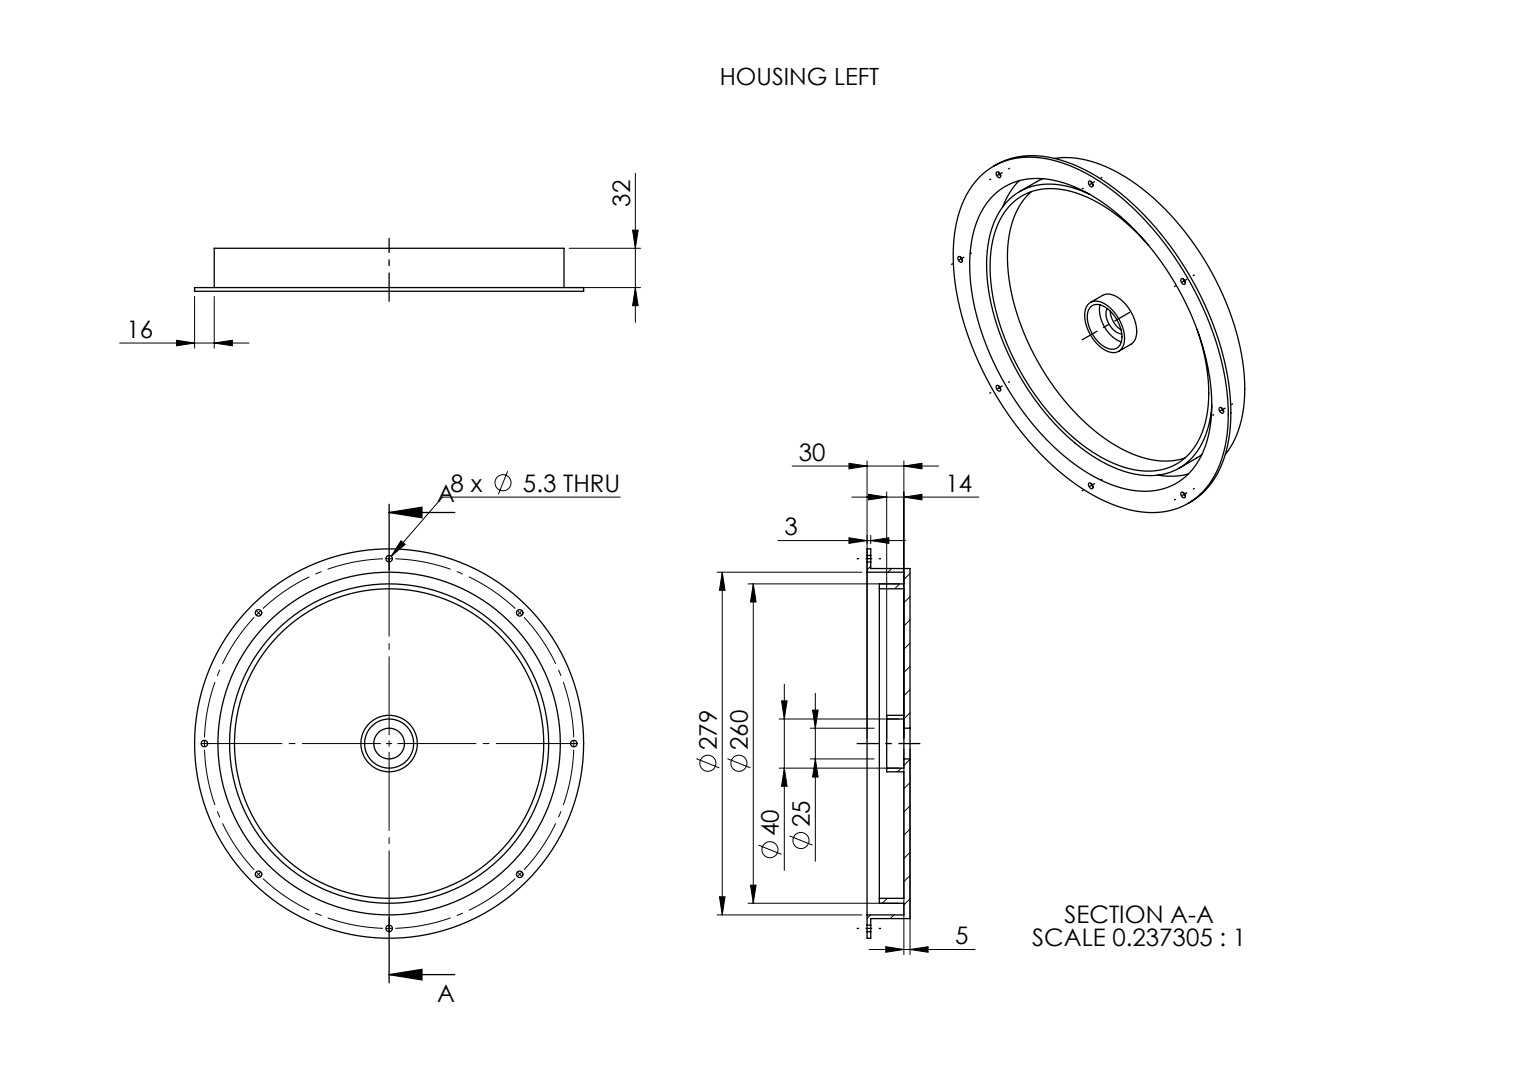
ISO-10303-21;
HEADER;
FILE_DESCRIPTION (('STEP AP214'),
    '1' );
FILE_NAME ('housing left.step',
    '2026-10-08T11:45:07',
    ( '' ),
    ( '' ),
    'SwSTEP 2.0',
    'SolidWorks 2026',
    '' );
FILE_SCHEMA (( 'AUTOMOTIVE_DESIGN' ));
ENDSEC;

DATA;
#75=EDGE_CURVE ( 'NONE', #34974, #23352, #8192, .T. ) ;
#80=DIRECTION ( 'NONE',  ( 1.000000000000000000, 0.000000000000000000, 0.000000000000000000 ) ) ;
#161=ADVANCED_FACE ( 'NONE', ( #9836 ), #29711, .F. ) ;
#175=EDGE_CURVE ( 'NONE', #28450, #28268, #33086, .T. ) ;
#184=DIRECTION ( 'NONE',  ( -0.2140725878556641593, -0.9768177553304296934, 0.000000000000000000 ) ) ;
#200=DIRECTION ( 'NONE',  ( -0.000000000000000000, -0.000000000000000000, 1.000000000000000000 ) ) ;
#245=ORIENTED_EDGE ( 'NONE', *, *, #22971, .F. ) ;
#258=DIRECTION ( 'NONE',  ( 1.000000000000000000, 0.000000000000000000, 0.000000000000000000 ) ) ;
#299=DIRECTION ( 'NONE',  ( 0.000000000000000000, 0.000000000000000000, 1.000000000000000000 ) ) ;
#312=CARTESIAN_POINT ( 'NONE',  ( -130.0000000000000284, 4.615443851143735910E-16, -20.00000000000000000 ) ) ;
#362=DIRECTION ( 'NONE',  ( 0.000000000000000000, 0.000000000000000000, 1.000000000000000000 ) ) ;
#399=CIRCLE ( 'NONE', #24866, 2.649999999999985700 ) ;
#444=EDGE_CURVE ( 'NONE', #11655, #6621, #32347, .T. ) ;
#503=PRESENTATION_STYLE_ASSIGNMENT (( #8148 ) ) ;
#513=ORIENTED_EDGE ( 'NONE', *, *, #20207, .F. ) ;
#609=ORIENTED_EDGE ( 'NONE', *, *, #444, .T. ) ;
#632=EDGE_CURVE ( 'NONE', #15962, #12068, #5869, .T. ) ;
#675=DIRECTION ( 'NONE',  ( 0.000000000000000000, 0.000000000000000000, 1.000000000000000000 ) ) ;
#711=( NAMED_UNIT ( * ) SI_UNIT ( $, .STERADIAN. ) SOLID_ANGLE_UNIT ( ) );
#788=EDGE_CURVE ( 'NONE', #6621, #11655, #5224, .T. ) ;
#808=ORIENTED_EDGE ( 'NONE', *, *, #27933, .T. ) ;
#847=FACE_BOUND ( 'NONE', #40043, .T. ) ;
#875=EDGE_LOOP ( 'NONE', ( #609, #11222 ) ) ;
#896=CARTESIAN_POINT ( 'NONE',  ( 109.0695705685763244, -106.4195705685744855, 6.999999999999998224 ) ) ;
#920=FACE_BOUND ( 'NONE', #14156, .T. ) ;
#939=CARTESIAN_POINT ( 'NONE',  ( -153.1500000000000057, -5.251434100941175950E-13, 9.999999999999998224 ) ) ;
#940=EDGE_CURVE ( 'NONE', #30306, #27122, #29838, .T. ) ;
#943=VECTOR ( 'NONE', #11137, 1000.000000000000000 ) ;
#945=CYLINDRICAL_SURFACE ( 'NONE', #19407, 126.0000000000000284 ) ;
#994=DIRECTION ( 'NONE',  ( 1.000000000000000000, 0.000000000000000000, 0.000000000000000000 ) ) ;
#1052=CARTESIAN_POINT ( 'NONE',  ( 5.657435538624008755E-15, 4.615443851143735910E-16, -20.00000000000001776 ) ) ;
#1084=CARTESIAN_POINT ( 'NONE',  ( 0.000000000000000000, 0.000000000000000000, -20.00000000000000000 ) ) ;
#1151=FACE_OUTER_BOUND ( 'NONE', #14974, .T. ) ;
#1244=AXIS2_PLACEMENT_3D ( 'NONE', #41617, #5610, #15672 ) ;
#1262=ORIENTED_EDGE ( 'NONE', *, *, #13717, .T. ) ;
#1270=DIRECTION ( 'NONE',  ( 1.000000000000000000, 0.000000000000000000, 0.000000000000000000 ) ) ;
#1292=ORIENTED_EDGE ( 'NONE', *, *, #35237, .T. ) ;
#1369=CARTESIAN_POINT ( 'NONE',  ( 106.4195705685741302, 106.4195705685767166, 6.999999999999998224 ) ) ;
#1372=( NAMED_UNIT ( * ) PLANE_ANGLE_UNIT ( ) SI_UNIT ( $, .RADIAN. ) );
#1390=DIRECTION ( 'NONE',  ( -0.000000000000000000, -0.000000000000000000, 1.000000000000000000 ) ) ;
#1393=FACE_BOUND ( 'NONE', #25323, .T. ) ;
#1394=DIRECTION ( 'NONE',  ( 1.000000000000000000, 0.000000000000000000, 0.000000000000000000 ) ) ;
#1439=ORIENTED_EDGE ( 'NONE', *, *, #28050, .T. ) ;
#1443=DIRECTION ( 'NONE',  ( 1.000000000000000000, 0.000000000000000000, 0.000000000000000000 ) ) ;
#1466=EDGE_CURVE ( 'NONE', #2965, #37680, #15217, .T. ) ;
#1475=CIRCLE ( 'NONE', #9143, 158.5000000000000284 ) ;
#1531=PRODUCT_CONTEXT ( 'NONE', #24534, 'mechanical' ) ;
#1567=CIRCLE ( 'NONE', #7140, 139.5000000000000000 ) ;
#1595=EDGE_CURVE ( 'NONE', #28016, #28450, #25874, .T. ) ;
#1638=CARTESIAN_POINT ( 'NONE',  ( 0.000000000000000000, 0.000000000000000000, 6.999999999999998224 ) ) ;
#1664=VERTEX_POINT ( 'NONE', #29142 ) ;
#1678=DIRECTION ( 'NONE',  ( 0.000000000000000000, 0.000000000000000000, 1.000000000000000000 ) ) ;
#1720=FACE_OUTER_BOUND ( 'NONE', #13675, .T. ) ;
#1744=CARTESIAN_POINT ( 'NONE',  ( 0.000000000000000000, 0.000000000000000000, -20.00000000000000000 ) ) ;
#1748=DIRECTION ( 'NONE',  ( 1.000000000000000000, 0.000000000000000000, 0.000000000000000000 ) ) ;
#1771=ORIENTED_EDGE ( 'NONE', *, *, #632, .T. ) ;
#1778=CARTESIAN_POINT ( 'NONE',  ( -139.5000000000000000, 0.000000000000000000, -20.00000000000000000 ) ) ;
#1886=CIRCLE ( 'NONE', #13069, 2.649999999999985700 ) ;
#1891=CARTESIAN_POINT ( 'NONE',  ( 0.000000000000000000, 0.000000000000000000, 6.999999999999998224 ) ) ;
#1951=AXIS2_PLACEMENT_3D ( 'NONE', #27384, #1390, #37822 ) ;
#2068=SURFACE_STYLE_USAGE ( .BOTH. , #26308 ) ;
#2083=VECTOR ( 'NONE', #34828, 1000.000000000000000 ) ;
#2084=CIRCLE ( 'NONE', #27888, 2.649999999999999467 ) ;
#2142=CARTESIAN_POINT ( 'NONE',  ( 0.000000000000000000, 0.000000000000000000, 9.999999999999998224 ) ) ;
#2145=ORIENTED_EDGE ( 'NONE', *, *, #7382, .T. ) ;
#2163=ORIENTED_EDGE ( 'NONE', *, *, #33430, .T. ) ;
#2172=AXIS2_PLACEMENT_3D ( 'NONE', #12279, #2402, #11860 ) ;
#2173=ORIENTED_EDGE ( 'NONE', *, *, #36590, .T. ) ;
#2189=ADVANCED_FACE ( 'NONE', ( #42996 ), #37911, .T. ) ;
#2226=DIRECTION ( 'NONE',  ( 1.000000000000000000, 0.000000000000000000, 0.000000000000000000 ) ) ;
#2259=DIRECTION ( 'NONE',  ( 0.000000000000000000, 0.000000000000000000, 1.000000000000000000 ) ) ;
#2305=EDGE_CURVE ( 'NONE', #20768, #38293, #28984, .T. ) ;
#2326=EDGE_LOOP ( 'NONE', ( #31321, #23179 ) ) ;
#2402=DIRECTION ( 'NONE',  ( 0.000000000000000000, 0.000000000000000000, 1.000000000000000000 ) ) ;
#2461=AXIS2_PLACEMENT_3D ( 'NONE', #39829, #23101, #19398 ) ;
#2472=CARTESIAN_POINT ( 'NONE',  ( 12.50000000000000000, 0.000000000000000000, -25.00000000000000000 ) ) ;
#2475=VERTEX_POINT ( 'NONE', #2950 ) ;
#2505=CYLINDRICAL_SURFACE ( 'NONE', #3072, 2.649999999999999467 ) ;
#2518=EDGE_CURVE ( 'NONE', #2965, #40561, #27577, .T. ) ;
#2556=LINE ( 'NONE', #43131, #13851 ) ;
#2582=VERTEX_POINT ( 'NONE', #3169 ) ;
#2584=CARTESIAN_POINT ( 'NONE',  ( 0.000000000000000000, -150.5000000000000284, 6.999999999999998224 ) ) ;
#2695=AXIS2_PLACEMENT_3D ( 'NONE', #14541, #21548, #27844 ) ;
#2713=DIRECTION ( 'NONE',  ( -0.000000000000000000, -0.000000000000000000, 1.000000000000000000 ) ) ;
#2721=ORIENTED_EDGE ( 'NONE', *, *, #75, .T. ) ;
#2788=CARTESIAN_POINT ( 'NONE',  ( 0.000000000000000000, 0.000000000000000000, 9.999999999999998224 ) ) ;
#2796=EDGE_CURVE ( 'NONE', #41293, #28005, #41533, .T. ) ;
#2831=DIRECTION ( 'NONE',  ( 1.000000000000000000, 0.000000000000000000, 0.000000000000000000 ) ) ;
#2877=DIRECTION ( 'NONE',  ( 1.000000000000000000, 0.000000000000000000, 0.000000000000000000 ) ) ;
#2904=DIRECTION ( 'NONE',  ( -0.000000000000000000, -0.000000000000000000, -1.000000000000000000 ) ) ;
#2926=CARTESIAN_POINT ( 'NONE',  ( 5.657435538624008755E-15, 4.615443851143735910E-16, 0.000000000000000000 ) ) ;
#2950=CARTESIAN_POINT ( 'NONE',  ( -109.0695705685756138, 106.4195705685752529, 6.999999999999998224 ) ) ;
#2965=VERTEX_POINT ( 'NONE', #39777 ) ;
#3029=FACE_OUTER_BOUND ( 'NONE', #8660, .T. ) ;
#3052=ADVANCED_BREP_SHAPE_REPRESENTATION ( '', ( #27661, #13552 ), #23961 ) ;
#3072=AXIS2_PLACEMENT_3D ( 'NONE', #19367, #2713, #18954 ) ;
#3088=ORIENTED_EDGE ( 'NONE', *, *, #34298, .T. ) ;
#3108=CARTESIAN_POINT ( 'NONE',  ( 150.5000000000000284, 1.576403824487674918E-12, 10.00000000000000000 ) ) ;
#3164=VERTEX_POINT ( 'NONE', #40215 ) ;
#3166=AXIS2_PLACEMENT_3D ( 'NONE', #30269, #27218, #33093 ) ;
#3169=CARTESIAN_POINT ( 'NONE',  ( 103.7695705685763556, -106.4195705685744855, 6.999999999999998224 ) ) ;
#3225=LINE ( 'NONE', #33785, #10904 ) ;
#3240=AXIS2_PLACEMENT_3D ( 'NONE', #12229, #24926, #42295 ) ;
#3260=CIRCLE ( 'NONE', #40212, 12.50000000000000000 ) ;
#3276=CARTESIAN_POINT ( 'NONE',  ( 126.0000000000000284, 1.589209405437102375E-14, -20.00000000000001776 ) ) ;
#3294=VECTOR ( 'NONE', #28045, 1000.000000000000000 ) ;
#3361=ORIENTED_EDGE ( 'NONE', *, *, #28288, .F. ) ;
#3447=VECTOR ( 'NONE', #13140, 1000.000000000000000 ) ;
#3488=FACE_OUTER_BOUND ( 'NONE', #19442, .T. ) ;
#3546=ORIENTED_EDGE ( 'NONE', *, *, #10588, .T. ) ;
#3569=VERTEX_POINT ( 'NONE', #20806 ) ;
#3594=CIRCLE ( 'NONE', #22478, 2.649999999999999467 ) ;
#3655=DIRECTION ( 'NONE',  ( 1.000000000000000000, 0.000000000000000000, 0.000000000000000000 ) ) ;
#3671=EDGE_LOOP ( 'NONE', ( #19488, #23768 ) ) ;
#3694=CARTESIAN_POINT ( 'NONE',  ( -150.5000000000000284, -5.254679414958916394E-13, 10.00000000000000000 ) ) ;
#3761=ORIENTED_EDGE ( 'NONE', *, *, #2518, .F. ) ;
#3767=DIRECTION ( 'NONE',  ( -0.000000000000000000, -0.000000000000000000, -1.000000000000000000 ) ) ;
#3782=DIRECTION ( 'NONE',  ( 0.000000000000000000, 0.000000000000000000, 1.000000000000000000 ) ) ;
#3821=AXIS2_PLACEMENT_3D ( 'NONE', #37877, #7998, #1443 ) ;
#3852=CARTESIAN_POINT ( 'NONE',  ( 0.000000000000000000, 0.000000000000000000, 0.000000000000000000 ) ) ;
#3942=VERTEX_POINT ( 'NONE', #32718 ) ;
#3945=CIRCLE ( 'NONE', #31183, 2.649999999999985700 ) ;
#3986=( NAMED_UNIT ( * ) SI_UNIT ( $, .STERADIAN. ) SOLID_ANGLE_UNIT ( ) );
#4187=EDGE_LOOP ( 'NONE', ( #28475, #30183, #13933, #34459 ) ) ;
#4292=CIRCLE ( 'NONE', #21782, 2.649999999999985700 ) ;
#4298=ORIENTED_EDGE ( 'NONE', *, *, #28288, .T. ) ;
#4317=CIRCLE ( 'NONE', #7824, 130.0000000000000284 ) ;
#4372=CARTESIAN_POINT ( 'NONE',  ( 150.5000000000000284, 1.576403824487674918E-12, 9.999999999999998224 ) ) ;
#4387=CARTESIAN_POINT ( 'NONE',  ( 0.000000000000000000, 0.000000000000000000, 9.999999999999998224 ) ) ;
#4555=CIRCLE ( 'NONE', #28979, 20.00000000000000000 ) ;
#4619=CARTESIAN_POINT ( 'NONE',  ( -2.649999999999987477, 150.5000000000000284, 10.00000000000000000 ) ) ;
#4648=( LENGTH_UNIT ( ) NAMED_UNIT ( * ) SI_UNIT ( .MILLI., .METRE. ) );
#4682=DIRECTION ( 'NONE',  ( -0.000000000000000000, -0.000000000000000000, 1.000000000000000000 ) ) ;
#4770=CARTESIAN_POINT ( 'NONE',  ( -103.7695705685756025, 106.4195705685752529, 6.999999999999998224 ) ) ;
#4831=CARTESIAN_POINT ( 'NONE',  ( 0.000000000000000000, 0.000000000000000000, -6.000000000000000000 ) ) ;
#4867=CARTESIAN_POINT ( 'NONE',  ( 0.000000000000000000, 0.000000000000000000, -25.00000000000000000 ) ) ;
#4995=DIRECTION ( 'NONE',  ( 0.000000000000000000, 0.000000000000000000, 1.000000000000000000 ) ) ;
#5016=VERTEX_POINT ( 'NONE', #15220 ) ;
#5024=AXIS2_PLACEMENT_3D ( 'NONE', #1084, #17511, #38393 ) ;
#5098=CYLINDRICAL_SURFACE ( 'NONE', #13103, 130.0000000000000284 ) ;
#5119=LINE ( 'NONE', #18713, #39076 ) ;
#5134=DIRECTION ( 'NONE',  ( 1.000000000000000000, 0.000000000000000000, 0.000000000000000000 ) ) ;
#5179=ORIENTED_EDGE ( 'NONE', *, *, #33784, .F. ) ;
#5213=VERTEX_POINT ( 'NONE', #39137 ) ;
#5224=CIRCLE ( 'NONE', #8679, 2.649999999999985700 ) ;
#5317=LINE ( 'NONE', #21528, #42896 ) ;
#5345=DIRECTION ( 'NONE',  ( -0.000000000000000000, -0.000000000000000000, 1.000000000000000000 ) ) ;
#5391=ORIENTED_EDGE ( 'NONE', *, *, #27933, .F. ) ;
#5468=ADVANCED_FACE ( 'NONE', ( #920, #8146 ), #40627, .F. ) ;
#5476=AXIS2_PLACEMENT_3D ( 'NONE', #21855, #25543, #42061 ) ;
#5493=ADVANCED_FACE ( 'NONE', ( #1151 ), #28023, .F. ) ;
#5594=PLANE ( 'NONE',  #34929 ) ;
#5610=DIRECTION ( 'NONE',  ( 0.000000000000000000, 0.000000000000000000, 1.000000000000000000 ) ) ;
#5644=DIRECTION ( 'NONE',  ( -1.000000000000000000, 0.000000000000000000, 0.000000000000000000 ) ) ;
#5674=ORIENTED_EDGE ( 'NONE', *, *, #18541, .F. ) ;
#5739=FACE_OUTER_BOUND ( 'NONE', #17879, .T. ) ;
#5869=CIRCLE ( 'NONE', #35146, 2.649999999999985700 ) ;
#5893=CIRCLE ( 'NONE', #40701, 2.649999999999985700 ) ;
#6004=AXIS2_PLACEMENT_3D ( 'NONE', #35091, #41640, #25530 ) ;
#6057=EDGE_LOOP ( 'NONE', ( #5391, #29218, #14335, #40689 ) ) ;
#6137=VECTOR ( 'NONE', #38491, 1000.000000000000000 ) ;
#6207=LINE ( 'NONE', #19553, #14969 ) ;
#6217=EDGE_CURVE ( 'NONE', #3164, #32065, #39038, .T. ) ;
#6364=EDGE_LOOP ( 'NONE', ( #10639, #808, #37020, #513 ) ) ;
#6427=DIRECTION ( 'NONE',  ( -0.000000000000000000, -0.000000000000000000, -1.000000000000000000 ) ) ;
#6507=ORIENTED_EDGE ( 'NONE', *, *, #22971, .T. ) ;
#6621=VERTEX_POINT ( 'NONE', #17369 ) ;
#6654=CARTESIAN_POINT ( 'NONE',  ( 0.000000000000000000, 0.000000000000000000, -20.00000000000000000 ) ) ;
#6679=ORIENTED_EDGE ( 'NONE', *, *, #36590, .F. ) ;
#6720=ADVANCED_FACE ( 'NONE', ( #27590 ), #15166, .F. ) ;
#6743=CIRCLE ( 'NONE', #30462, 158.5000000000000284 ) ;
#6764=DIRECTION ( 'NONE',  ( 1.000000000000000000, 0.000000000000000000, 0.000000000000000000 ) ) ;
#6777=AXIS2_PLACEMENT_3D ( 'NONE', #12751, #29978, #2877 ) ;
#6785=DIRECTION ( 'NONE',  ( 0.000000000000000000, 0.000000000000000000, 1.000000000000000000 ) ) ;
#6787=PLANE ( 'NONE',  #10176 ) ;
#6910=ADVANCED_FACE ( 'NONE', ( #9212 ), #18676, .F. ) ;
#6987=CARTESIAN_POINT ( 'NONE',  ( 20.00000000000000000, 2.449293598294706513E-15, -20.00000000000000000 ) ) ;
#7016=EDGE_LOOP ( 'NONE', ( #20071, #3761, #31295, #27188 ) ) ;
#7018=CARTESIAN_POINT ( 'NONE',  ( 5.657435538624008755E-15, 4.615443851143735910E-16, 367.6955262170047263 ) ) ;
#7051=CARTESIAN_POINT ( 'NONE',  ( 126.0000000000000284, 1.589209405437102375E-14, 0.000000000000000000 ) ) ;
#7076=CARTESIAN_POINT ( 'NONE',  ( 0.000000000000000000, 0.000000000000000000, -20.00000000000000000 ) ) ;
#7140=AXIS2_PLACEMENT_3D ( 'NONE', #1744, #8084, #37747 ) ;
#7184=CARTESIAN_POINT ( 'NONE',  ( 0.000000000000000000, 0.000000000000000000, -25.00000000000000000 ) ) ;
#7230=CYLINDRICAL_SURFACE ( 'NONE', #42624, 12.50000000000000000 ) ;
#7288=DIRECTION ( 'NONE',  ( 0.000000000000000000, 0.000000000000000000, 1.000000000000000000 ) ) ;
#7324=AXIS2_PLACEMENT_3D ( 'NONE', #19545, #16050, #19335 ) ;
#7325=EDGE_LOOP ( 'NONE', ( #19158, #18409 ) ) ;
#7345=ORIENTED_EDGE ( 'NONE', *, *, #16067, .T. ) ;
#7349=EDGE_CURVE ( 'NONE', #2475, #5016, #19890, .T. ) ;
#7365=AXIS2_PLACEMENT_3D ( 'NONE', #33738, #23312, #43123 ) ;
#7382=EDGE_CURVE ( 'NONE', #38293, #23352, #26309, .T. ) ;
#7412=EDGE_LOOP ( 'NONE', ( #17057, #36600 ) ) ;
#7425=CARTESIAN_POINT ( 'NONE',  ( 2.649999999999987477, -150.5000000000000284, 10.00000000000000000 ) ) ;
#7434=AXIS2_PLACEMENT_3D ( 'NONE', #40284, #29687, #25987 ) ;
#7471=DIRECTION ( 'NONE',  ( 0.000000000000000000, 0.000000000000000000, 1.000000000000000000 ) ) ;
#7474=ORIENTED_EDGE ( 'NONE', *, *, #25003, .T. ) ;
#7531=EDGE_LOOP ( 'NONE', ( #41415, #27687, #7686, #2145 ) ) ;
#7538=CARTESIAN_POINT ( 'NONE',  ( 147.8500000000000227, 1.576728355889448963E-12, 10.00000000000000000 ) ) ;
#7557=CIRCLE ( 'NONE', #26359, 2.649999999999993694 ) ;
#7686=ORIENTED_EDGE ( 'NONE', *, *, #2305, .T. ) ;
#7694=ORIENTED_EDGE ( 'NONE', *, *, #14997, .F. ) ;
#7706=LINE ( 'NONE', #10554, #42197 ) ;
#7709=( NAMED_UNIT ( * ) PLANE_ANGLE_UNIT ( ) SI_UNIT ( $, .RADIAN. ) );
#7723=DIRECTION ( 'NONE',  ( -0.000000000000000000, -0.000000000000000000, -1.000000000000000000 ) ) ;
#7724=DIRECTION ( 'NONE',  ( 1.000000000000000000, 0.000000000000000000, 0.000000000000000000 ) ) ;
#7728=DIRECTION ( 'NONE',  ( -0.000000000000000000, -0.000000000000000000, -1.000000000000000000 ) ) ;
#7731=AXIS2_PLACEMENT_3D ( 'NONE', #19976, #10765, #37371 ) ;
#7745=DIRECTION ( 'NONE',  ( -1.000000000000000000, 0.000000000000000000, 0.000000000000000000 ) ) ;
#7824=AXIS2_PLACEMENT_3D ( 'NONE', #33782, #29898, #3655 ) ;
#7826=VERTEX_POINT ( 'NONE', #9568 ) ;
#7842=DIRECTION ( 'NONE',  ( -0.2140725878556641315, -0.9768177553304295824, 0.000000000000000000 ) ) ;
#7908=AXIS2_PLACEMENT_3D ( 'NONE', #29094, #22149, #16213 ) ;
#7914=DIRECTION ( 'NONE',  ( 0.000000000000000000, 0.000000000000000000, 1.000000000000000000 ) ) ;
#7943=DIRECTION ( 'NONE',  ( 0.000000000000000000, 0.000000000000000000, 1.000000000000000000 ) ) ;
#7998=DIRECTION ( 'NONE',  ( -0.000000000000000000, -0.000000000000000000, 1.000000000000000000 ) ) ;
#8081=PLANE ( 'NONE',  #5024 ) ;
#8084=DIRECTION ( 'NONE',  ( -0.000000000000000000, -0.000000000000000000, -1.000000000000000000 ) ) ;
#8090=CARTESIAN_POINT ( 'NONE',  ( 106.4195705685763471, -106.4195705685744855, 10.00000000000000000 ) ) ;
#8146=FACE_OUTER_BOUND ( 'NONE', #40371, .T. ) ;
#8148=SURFACE_STYLE_USAGE ( .BOTH. , #11433 ) ;
#8184=DIRECTION ( 'NONE',  ( -0.000000000000000000, -0.000000000000000000, -1.000000000000000000 ) ) ;
#8192=LINE ( 'NONE', #22547, #31702 ) ;
#8209=EDGE_CURVE ( 'NONE', #11655, #16140, #8235, .T. ) ;
#8223=CARTESIAN_POINT ( 'NONE',  ( 103.7695705685741387, 106.4195705685767166, 9.999999999999998224 ) ) ;
#8231=DIRECTION ( 'NONE',  ( -0.000000000000000000, -0.000000000000000000, 1.000000000000000000 ) ) ;
#8235=LINE ( 'NONE', #11750, #32805 ) ;
#8264=CYLINDRICAL_SURFACE ( 'NONE', #32930, 23.00000000000000000 ) ;
#8293=ORIENTED_EDGE ( 'NONE', *, *, #8555, .T. ) ;
#8307=ADVANCED_FACE ( 'NONE', ( #36115, #22864, #25905, #35681, #19369, #42866, #38957, #15649, #19576, #12381 ), #5594, .T. ) ;
#8310=SHAPE_DEFINITION_REPRESENTATION ( #9548, #39082 ) ;
#8349=ORIENTED_EDGE ( 'NONE', *, *, #30164, .T. ) ;
#8374=EDGE_CURVE ( 'NONE', #37517, #41239, #41167, .T. ) ;
#8432=VERTEX_POINT ( 'NONE', #9927 ) ;
#8469=DIRECTION ( 'NONE',  ( -1.000000000000000000, 0.000000000000000000, 0.000000000000000000 ) ) ;
#8490=FACE_OUTER_BOUND ( 'NONE', #6364, .T. ) ;
#8517=VECTOR ( 'NONE', #35103, 1000.000000000000000 ) ;
#8533=EDGE_LOOP ( 'NONE', ( #21293, #11741, #40964, #39910 ) ) ;
#8551=ORIENTED_EDGE ( 'NONE', *, *, #788, .F. ) ;
#8555=EDGE_CURVE ( 'NONE', #19787, #10716, #29372, .T. ) ;
#8565=ORIENTED_EDGE ( 'NONE', *, *, #34904, .F. ) ;
#8660=EDGE_LOOP ( 'NONE', ( #33670, #37022, #26076, #245 ) ) ;
#8679=AXIS2_PLACEMENT_3D ( 'NONE', #29666, #42940, #26395 ) ;
#8796=EDGE_CURVE ( 'NONE', #38324, #36435, #4292, .T. ) ;
#8830=ORIENTED_EDGE ( 'NONE', *, *, #24249, .T. ) ;
#8839=EDGE_LOOP ( 'NONE', ( #40459, #2721, #35422, #10366 ) ) ;
#8852=CIRCLE ( 'NONE', #3240, 2.649999999999987477 ) ;
#8879=ORIENTED_EDGE ( 'NONE', *, *, #36479, .F. ) ;
#8905=VECTOR ( 'NONE', #17273, 1000.000000000000000 ) ;
#8919=PLANE ( 'NONE',  #35283 ) ;
#8933=LINE ( 'NONE', #32060, #8517 ) ;
#8965=EDGE_CURVE ( 'NONE', #2475, #25511, #3594, .T. ) ;
#8993=CIRCLE ( 'NONE', #16692, 139.5000000000000000 ) ;
#9035=EDGE_LOOP ( 'NONE', ( #8293, #8349 ) ) ;
#9037=EDGE_CURVE ( 'NONE', #22117, #28268, #8933, .T. ) ;
#9039=FACE_BOUND ( 'NONE', #21670, .T. ) ;
#9141=FACE_OUTER_BOUND ( 'NONE', #42367, .T. ) ;
#9143=AXIS2_PLACEMENT_3D ( 'NONE', #2788, #12871, #22502 ) ;
#9146=DIRECTION ( 'NONE',  ( 1.000000000000000000, 0.000000000000000000, 0.000000000000000000 ) ) ;
#9170=AXIS2_PLACEMENT_3D ( 'NONE', #24435, #11320, #23998 ) ;
#9175=CARTESIAN_POINT ( 'NONE',  ( 0.000000000000000000, 150.5000000000000284, 10.00000000000000000 ) ) ;
#9185=DIRECTION ( 'NONE',  ( 1.000000000000000000, 0.000000000000000000, 0.000000000000000000 ) ) ;
#9212=FACE_OUTER_BOUND ( 'NONE', #26209, .T. ) ;
#9242=FACE_OUTER_BOUND ( 'NONE', #8839, .T. ) ;
#9269=VERTEX_POINT ( 'NONE', #32695 ) ;
#9270=DIRECTION ( 'NONE',  ( -0.000000000000000000, -0.000000000000000000, 1.000000000000000000 ) ) ;
#9272=EDGE_CURVE ( 'NONE', #37517, #39291, #36171, .T. ) ;
#9380=CARTESIAN_POINT ( 'NONE',  ( -109.0695705685756138, 106.4195705685752529, 9.999999999999998224 ) ) ;
#9431=VECTOR ( 'NONE', #11247, 1000.000000000000000 ) ;
#9476=LINE ( 'NONE', #2472, #27599 ) ;
#9490=EDGE_CURVE ( 'NONE', #12068, #15962, #25975, .T. ) ;
#9509=CARTESIAN_POINT ( 'NONE',  ( -2.649999999999993694, 150.5000000000000284, 6.999999999999998224 ) ) ;
#9548=PRODUCT_DEFINITION_SHAPE ( 'NONE', 'NONE',  #35852 ) ;
#9556=LINE ( 'NONE', #15917, #18343 ) ;
#9561=AXIS2_PLACEMENT_3D ( 'NONE', #22432, #41811, #11958 ) ;
#9568=CARTESIAN_POINT ( 'NONE',  ( 23.00000000000000000, 2.816687638038912352E-15, -6.000000000000000000 ) ) ;
#9596=CARTESIAN_POINT ( 'NONE',  ( 0.000000000000000000, -150.5000000000000284, 9.999999999999998224 ) ) ;
#9620=AXIS2_PLACEMENT_3D ( 'NONE', #7076, #10578, #31307 ) ;
#9670=ADVANCED_FACE ( 'NONE', ( #34629 ), #24424, .T. ) ;
#9800=DIRECTION ( 'NONE',  ( 1.000000000000000000, 0.000000000000000000, 0.000000000000000000 ) ) ;
#9823=EDGE_LOOP ( 'NONE', ( #26961, #29977, #17627, #22621 ) ) ;
#9836=FACE_OUTER_BOUND ( 'NONE', #31839, .T. ) ;
#9927=CARTESIAN_POINT ( 'NONE',  ( 103.7695705685741387, 106.4195705685767166, 6.999999999999998224 ) ) ;
#9959=ORIENTED_EDGE ( 'NONE', *, *, #12072, .T. ) ;
#10001=MECHANICAL_DESIGN_GEOMETRIC_PRESENTATION_REPRESENTATION('',(#17715),#37156);
#10052=DIRECTION ( 'NONE',  ( 1.000000000000000000, 0.000000000000000000, 0.000000000000000000 ) ) ;
#10176=AXIS2_PLACEMENT_3D ( 'NONE', #17306, #40366, #40147 ) ;
#10213=DIRECTION ( 'NONE',  ( 1.000000000000000000, 0.000000000000000000, 0.000000000000000000 ) ) ;
#10250=LINE ( 'NONE', #30766, #39930 ) ;
#10264=CARTESIAN_POINT ( 'NONE',  ( -139.5000000000000000, 0.000000000000000000, 9.999999999999998224 ) ) ;
#10328=ORIENTED_EDGE ( 'NONE', *, *, #15054, .F. ) ;
#10366=ORIENTED_EDGE ( 'NONE', *, *, #2305, .F. ) ;
#10496=FACE_OUTER_BOUND ( 'NONE', #39299, .T. ) ;
#10523=ORIENTED_EDGE ( 'NONE', *, *, #13430, .F. ) ;
#10551=VECTOR ( 'NONE', #35339, 1000.000000000000000 ) ;
#10554=CARTESIAN_POINT ( 'NONE',  ( 158.5000000000000284, 0.000000000000000000, 6.999999999999998224 ) ) ;
#10558=FILL_AREA_STYLE_COLOUR ( '', #23278 ) ;
#10578=DIRECTION ( 'NONE',  ( 0.000000000000000000, 0.000000000000000000, 1.000000000000000000 ) ) ;
#10588=EDGE_CURVE ( 'NONE', #36784, #9269, #30759, .T. ) ;
#10615=ORIENTED_EDGE ( 'NONE', *, *, #16067, .F. ) ;
#10639=ORIENTED_EDGE ( 'NONE', *, *, #9490, .F. ) ;
#10681=LINE ( 'NONE', #27719, #8905 ) ;
#10696=CARTESIAN_POINT ( 'NONE',  ( 153.1500000000000057, 1.576403824487674918E-12, 10.00000000000000000 ) ) ;
#10699=DIRECTION ( 'NONE',  ( -0.000000000000000000, -0.000000000000000000, -1.000000000000000000 ) ) ;
#10704=ORIENTED_EDGE ( 'NONE', *, *, #11733, .F. ) ;
#10716=VERTEX_POINT ( 'NONE', #6987 ) ;
#10765=DIRECTION ( 'NONE',  ( 0.000000000000000000, 0.000000000000000000, 1.000000000000000000 ) ) ;
#10767=ORIENTED_EDGE ( 'NONE', *, *, #37473, .T. ) ;
#10786=CARTESIAN_POINT ( 'NONE',  ( -103.7695705685756167, 106.4195705685752529, 10.00000000000000000 ) ) ;
#10817=VECTOR ( 'NONE', #38137, 1000.000000000000000 ) ;
#10904=VECTOR ( 'NONE', #23355, 1000.000000000000000 ) ;
#10917=ORIENTED_EDGE ( 'NONE', *, *, #40006, .F. ) ;
#10938=DIRECTION ( 'NONE',  ( 1.000000000000000000, 0.000000000000000000, 0.000000000000000000 ) ) ;
#10945=AXIS2_PLACEMENT_3D ( 'NONE', #7018, #43017, #13825 ) ;
#10979=AXIS2_PLACEMENT_3D ( 'NONE', #21319, #4682, #21753 ) ;
#11137=DIRECTION ( 'NONE',  ( -0.000000000000000000, -0.000000000000000000, 1.000000000000000000 ) ) ;
#11150=FACE_OUTER_BOUND ( 'NONE', #25415, .T. ) ;
#11185=AXIS2_PLACEMENT_3D ( 'NONE', #9175, #26202, #39051 ) ;
#11222=ORIENTED_EDGE ( 'NONE', *, *, #788, .T. ) ;
#11237=ORIENTED_EDGE ( 'NONE', *, *, #175, .F. ) ;
#11247=DIRECTION ( 'NONE',  ( -0.000000000000000000, -0.000000000000000000, -1.000000000000000000 ) ) ;
#11261=VERTEX_POINT ( 'NONE', #36988 ) ;
#11281=CARTESIAN_POINT ( 'NONE',  ( -2.649999999999987477, -150.5000000000000284, 10.00000000000000000 ) ) ;
#11301=AXIS2_PLACEMENT_3D ( 'NONE', #3694, #17072, #10052 ) ;
#11320=DIRECTION ( 'NONE',  ( 0.000000000000000000, 0.000000000000000000, 1.000000000000000000 ) ) ;
#11362=DIRECTION ( 'NONE',  ( 0.000000000000000000, 0.000000000000000000, 1.000000000000000000 ) ) ;
#11371=AXIS2_PLACEMENT_3D ( 'NONE', #9596, #36190, #22085 ) ;
#11433=SURFACE_SIDE_STYLE ('',( #37593 ) ) ;
#11455=ORIENTED_EDGE ( 'NONE', *, *, #8374, .T. ) ;
#11467=CYLINDRICAL_SURFACE ( 'NONE', #39639, 139.5000000000000000 ) ;
#11487=ORIENTED_EDGE ( 'NONE', *, *, #40914, .T. ) ;
#11561=CIRCLE ( 'NONE', #17149, 2.649999999999985700 ) ;
#11614=ADVANCED_FACE ( 'NONE', ( #23856 ), #7230, .F. ) ;
#11655=VERTEX_POINT ( 'NONE', #15338 ) ;
#11671=DIRECTION ( 'NONE',  ( -0.000000000000000000, -0.000000000000000000, 1.000000000000000000 ) ) ;
#11684=PLANE ( 'NONE',  #13759 ) ;
#11691=DIRECTION ( 'NONE',  ( -0.000000000000000000, -0.000000000000000000, 1.000000000000000000 ) ) ;
#11733=EDGE_CURVE ( 'NONE', #6621, #39372, #9556, .T. ) ;
#11737=ADVANCED_FACE ( 'NONE', ( #22471 ), #22911, .F. ) ;
#11740=AXIS2_PLACEMENT_3D ( 'NONE', #4867, #14501, #21510 ) ;
#11741=ORIENTED_EDGE ( 'NONE', *, *, #40550, .T. ) ;
#11750=CARTESIAN_POINT ( 'NONE',  ( 153.1500000000000057, 1.576403824487674918E-12, 9.999999999999998224 ) ) ;
#11860=DIRECTION ( 'NONE',  ( 1.000000000000000000, 0.000000000000000000, 0.000000000000000000 ) ) ;
#11893=ORIENTED_EDGE ( 'NONE', *, *, #16787, .T. ) ;
#11958=DIRECTION ( 'NONE',  ( 1.000000000000000000, 0.000000000000000000, 0.000000000000000000 ) ) ;
#11999=FACE_BOUND ( 'NONE', #2326, .T. ) ;
#12011=DIRECTION ( 'NONE',  ( -0.000000000000000000, -0.000000000000000000, 1.000000000000000000 ) ) ;
#12068=VERTEX_POINT ( 'NONE', #41797 ) ;
#12072=EDGE_CURVE ( 'NONE', #8432, #38324, #21359, .T. ) ;
#12100=EDGE_CURVE ( 'NONE', #39291, #24752, #22323, .T. ) ;
#12107=DIRECTION ( 'NONE',  ( 1.000000000000000000, 0.000000000000000000, -0.000000000000000000 ) ) ;
#12136=DIRECTION ( 'NONE',  ( 0.000000000000000000, 0.000000000000000000, 1.000000000000000000 ) ) ;
#12163=DIRECTION ( 'NONE',  ( 1.000000000000000000, 0.000000000000000000, -0.000000000000000000 ) ) ;
#12166=AXIS2_PLACEMENT_3D ( 'NONE', #15515, #21655, #9146 ) ;
#12229=CARTESIAN_POINT ( 'NONE',  ( 0.000000000000000000, -150.5000000000000284, 10.00000000000000000 ) ) ;
#12247=AXIS2_PLACEMENT_3D ( 'NONE', #41980, #2259, #42188 ) ;
#12268=ORIENTED_EDGE ( 'NONE', *, *, #33800, .T. ) ;
#12273=ORIENTED_EDGE ( 'NONE', *, *, #16870, .T. ) ;
#12279=CARTESIAN_POINT ( 'NONE',  ( 0.000000000000000000, 0.000000000000000000, -20.00000000000000000 ) ) ;
#12318=DIRECTION ( 'NONE',  ( 0.000000000000000000, 0.000000000000000000, 1.000000000000000000 ) ) ;
#12329=ORIENTED_EDGE ( 'NONE', *, *, #37504, .T. ) ;
#12340=FACE_BOUND ( 'NONE', #37292, .T. ) ;
#12381=FACE_OUTER_BOUND ( 'NONE', #16135, .T. ) ;
#12426=ORIENTED_EDGE ( 'NONE', *, *, #11733, .T. ) ;
#12427=DIRECTION ( 'NONE',  ( 1.000000000000000000, 0.000000000000000000, -0.000000000000000000 ) ) ;
#12488=DIRECTION ( 'NONE',  ( -0.000000000000000000, -0.000000000000000000, -1.000000000000000000 ) ) ;
#12516=ORIENTED_EDGE ( 'NONE', *, *, #1595, .F. ) ;
#12652=AXIS2_PLACEMENT_3D ( 'NONE', #2584, #42513, #25966 ) ;
#12657=EDGE_LOOP ( 'NONE', ( #41920, #30224 ) ) ;
#12695=ORIENTED_EDGE ( 'NONE', *, *, #9272, .F. ) ;
#12728=ORIENTED_EDGE ( 'NONE', *, *, #41786, .T. ) ;
#12751=CARTESIAN_POINT ( 'NONE',  ( 0.000000000000000000, 150.5000000000000284, 9.999999999999998224 ) ) ;
#12781=LINE ( 'NONE', #39149, #26911 ) ;
#12836=AXIS2_PLACEMENT_3D ( 'NONE', #25553, #38176, #21649 ) ;
#12871=DIRECTION ( 'NONE',  ( 0.000000000000000000, 0.000000000000000000, 1.000000000000000000 ) ) ;
#13005=FILL_AREA_STYLE ('',( #38725 ) ) ;
#13069=AXIS2_PLACEMENT_3D ( 'NONE', #32531, #35774, #9185 ) ;
#13091=ORIENTED_EDGE ( 'NONE', *, *, #13893, .F. ) ;
#13103=AXIS2_PLACEMENT_3D ( 'NONE', #35620, #15591, #38902 ) ;
#13134=AXIS2_PLACEMENT_3D ( 'NONE', #7184, #20542, #6764 ) ;
#13140=DIRECTION ( 'NONE',  ( -0.000000000000000000, -0.000000000000000000, -1.000000000000000000 ) ) ;
#13185=ORIENTED_EDGE ( 'NONE', *, *, #24368, .T. ) ;
#13309=DIRECTION ( 'NONE',  ( -0.000000000000000000, -0.000000000000000000, -1.000000000000000000 ) ) ;
#13349=EDGE_LOOP ( 'NONE', ( #31149, #13185, #13687, #38615 ) ) ;
#13430=EDGE_CURVE ( 'NONE', #41700, #20548, #34528, .T. ) ;
#13473=ORIENTED_EDGE ( 'NONE', *, *, #17637, .F. ) ;
#13527=LINE ( 'NONE', #27053, #19992 ) ;
#13552=AXIS2_PLACEMENT_3D ( 'NONE', #3852, #14597, #10213 ) ;
#13612=ORIENTED_EDGE ( 'NONE', *, *, #40914, .F. ) ;
#13675=EDGE_LOOP ( 'NONE', ( #29104, #14821, #36892, #1262 ) ) ;
#13687=ORIENTED_EDGE ( 'NONE', *, *, #6217, .T. ) ;
#13717=EDGE_CURVE ( 'NONE', #23467, #30139, #28344, .T. ) ;
#13759=AXIS2_PLACEMENT_3D ( 'NONE', #37825, #7943, #12107 ) ;
#13825=DIRECTION ( 'NONE',  ( -1.000000000000000000, 0.000000000000000000, 0.000000000000000000 ) ) ;
#13851=VECTOR ( 'NONE', #29425, 1000.000000000000000 ) ;
#13882=DIRECTION ( 'NONE',  ( 0.000000000000000000, 0.000000000000000000, 1.000000000000000000 ) ) ;
#13889=CARTESIAN_POINT ( 'NONE',  ( 106.4195705685763471, -106.4195705685744855, 6.999999999999998224 ) ) ;
#13893=EDGE_CURVE ( 'NONE', #39372, #16140, #27642, .T. ) ;
#13933=ORIENTED_EDGE ( 'NONE', *, *, #22030, .T. ) ;
#13940=ORIENTED_EDGE ( 'NONE', *, *, #15058, .F. ) ;
#14061=PLANE ( 'NONE',  #7731 ) ;
#14067=CYLINDRICAL_SURFACE ( 'NONE', #39827, 2.649999999999985700 ) ;
#14072=SHAPE_REPRESENTATION_RELATIONSHIP ( 'NONE' , 'NONE' ,  #39082, #3052 ) ;
#14081=ORIENTED_EDGE ( 'NONE', *, *, #2796, .F. ) ;
#14101=EDGE_LOOP ( 'NONE', ( #17500, #10523 ) ) ;
#14132=EDGE_LOOP ( 'NONE', ( #37286, #3361 ) ) ;
#14156=EDGE_LOOP ( 'NONE', ( #39555, #2163 ) ) ;
#14335=ORIENTED_EDGE ( 'NONE', *, *, #20207, .T. ) ;
#14361=DIRECTION ( 'NONE',  ( -0.000000000000000000, -0.000000000000000000, 1.000000000000000000 ) ) ;
#14387=ADVANCED_FACE ( 'NONE', ( #29051 ), #35987, .F. ) ;
#14491=CARTESIAN_POINT ( 'NONE',  ( 103.7695705685763556, -106.4195705685744855, 10.00000000000000000 ) ) ;
#14501=DIRECTION ( 'NONE',  ( 0.000000000000000000, 0.000000000000000000, 1.000000000000000000 ) ) ;
#14510=DIRECTION ( 'NONE',  ( 1.000000000000000000, 0.000000000000000000, 0.000000000000000000 ) ) ;
#14541=CARTESIAN_POINT ( 'NONE',  ( 0.000000000000000000, 150.5000000000000284, 6.999999999999998224 ) ) ;
#14554=ORIENTED_EDGE ( 'NONE', *, *, #33381, .F. ) ;
#14594=DIRECTION ( 'NONE',  ( 1.000000000000000000, 0.000000000000000000, 0.000000000000000000 ) ) ;
#14597=DIRECTION ( 'NONE',  ( 0.000000000000000000, 0.000000000000000000, 1.000000000000000000 ) ) ;
#14601=CARTESIAN_POINT ( 'NONE',  ( -106.4195705685756081, 106.4195705685752529, 10.00000000000000000 ) ) ;
#14602=ORIENTED_EDGE ( 'NONE', *, *, #21778, .T. ) ;
#14660=FACE_OUTER_BOUND ( 'NONE', #14132, .T. ) ;
#14727=CARTESIAN_POINT ( 'NONE',  ( 106.4195705685741302, 106.4195705685767166, 9.999999999999998224 ) ) ;
#14755=VERTEX_POINT ( 'NONE', #41584 ) ;
#14821=ORIENTED_EDGE ( 'NONE', *, *, #19612, .T. ) ;
#14891=DIRECTION ( 'NONE',  ( 1.000000000000000000, 0.000000000000000000, 0.000000000000000000 ) ) ;
#14957=CARTESIAN_POINT ( 'NONE',  ( -106.4195705685748550, -106.4195705685759776, 9.999999999999998224 ) ) ;
#14969=VECTOR ( 'NONE', #2904, 1000.000000000000000 ) ;
#14974=EDGE_LOOP ( 'NONE', ( #11455, #10767, #4298, #12695 ) ) ;
#14989=VERTEX_POINT ( 'NONE', #17809 ) ;
#14997=EDGE_CURVE ( 'NONE', #9269, #36784, #16605, .T. ) ;
#15054=EDGE_CURVE ( 'NONE', #34854, #10716, #24570, .T. ) ;
#15058=EDGE_CURVE ( 'NONE', #37680, #16448, #34007, .T. ) ;
#15086=VERTEX_POINT ( 'NONE', #34340 ) ;
#15134=ADVANCED_FACE ( 'NONE', ( #27173 ), #945, .F. ) ;
#15166=CYLINDRICAL_SURFACE ( 'NONE', #36676, 2.649999999999985700 ) ;
#15174=ORIENTED_EDGE ( 'NONE', *, *, #16894, .F. ) ;
#15191=ADVANCED_FACE ( 'NONE', ( #31951 ), #38467, .F. ) ;
#15207=ADVANCED_FACE ( 'NONE', ( #5739 ), #25644, .T. ) ;
#15217=LINE ( 'NONE', #31111, #6137 ) ;
#15220=CARTESIAN_POINT ( 'NONE',  ( -109.0695705685755996, 106.4195705685752529, 10.00000000000000000 ) ) ;
#15229=ADVANCED_FACE ( 'NONE', ( #21532 ), #5098, .T. ) ;
#15259=DIRECTION ( 'NONE',  ( 0.000000000000000000, 0.000000000000000000, 1.000000000000000000 ) ) ;
#15280=CARTESIAN_POINT ( 'NONE',  ( 2.649999999999993694, 150.5000000000000284, 9.999999999999998224 ) ) ;
#15321=EDGE_LOOP ( 'NONE', ( #7474, #38475, #12728, #13473 ) ) ;
#15337=CARTESIAN_POINT ( 'NONE',  ( -158.5000000000000284, 1.941065176648555254E-14, 9.999999999999998224 ) ) ;
#15338=CARTESIAN_POINT ( 'NONE',  ( 153.1500000000000057, 1.576403824487674918E-12, 6.999999999999998224 ) ) ;
#15353=APPLICATION_CONTEXT ( 'automotive_design' ) ;
#15515=CARTESIAN_POINT ( 'NONE',  ( 150.5000000000000284, 1.576403824487674918E-12, 6.999999999999998224 ) ) ;
#15553=DIRECTION ( 'NONE',  ( 1.000000000000000000, 0.000000000000000000, 0.000000000000000000 ) ) ;
#15579=ORIENTED_EDGE ( 'NONE', *, *, #18893, .T. ) ;
#15591=DIRECTION ( 'NONE',  ( -0.000000000000000000, -0.000000000000000000, -1.000000000000000000 ) ) ;
#15595=CARTESIAN_POINT ( 'NONE',  ( 139.5000000000000000, 1.708382284810557841E-14, 9.999999999999998224 ) ) ;
#15600=CARTESIAN_POINT ( 'NONE',  ( 0.000000000000000000, 150.5000000000000284, 10.00000000000000000 ) ) ;
#15615=CARTESIAN_POINT ( 'NONE',  ( -142.5000000000000284, 1.745121688784978386E-14, -25.00000000000000000 ) ) ;
#15649=FACE_BOUND ( 'NONE', #12657, .T. ) ;
#15672=DIRECTION ( 'NONE',  ( 1.000000000000000000, 0.000000000000000000, 0.000000000000000000 ) ) ;
#15694=COLOUR_RGB ( '', 0.09019608, 0.27058824, 0.51372549) ;
#15720=EDGE_LOOP ( 'NONE', ( #16663, #10615 ) ) ;
#15782=AXIS2_PLACEMENT_3D ( 'NONE', #23401, #17512, #21013 ) ;
#15801=CIRCLE ( 'NONE', #31116, 12.50000000000000000 ) ;
#15812=EDGE_CURVE ( 'NONE', #36979, #20273, #3260, .T. ) ;
#15827=FACE_BOUND ( 'NONE', #16750, .T. ) ;
#15894=CARTESIAN_POINT ( 'NONE',  ( 0.000000000000000000, 0.000000000000000000, -25.00000000000000000 ) ) ;
#15917=CARTESIAN_POINT ( 'NONE',  ( 147.8500000000000227, 1.576728355889448963E-12, 9.999999999999998224 ) ) ;
#15932=DIRECTION ( 'NONE',  ( -0.000000000000000000, -0.000000000000000000, -1.000000000000000000 ) ) ;
#15933=AXIS2_PLACEMENT_3D ( 'NONE', #37080, #30127, #184 ) ;
#15949=UNCERTAINTY_MEASURE_WITH_UNIT (LENGTH_MEASURE( 1.000000000000000082E-05 ), #20629, 'distance_accuracy_value', 'NONE');
#15962=VERTEX_POINT ( 'NONE', #28905 ) ;
#16050=DIRECTION ( 'NONE',  ( 0.000000000000000000, 0.000000000000000000, 1.000000000000000000 ) ) ;
#16060=ADVANCED_FACE ( 'NONE', ( #3029 ), #30135, .F. ) ;
#16067=EDGE_CURVE ( 'NONE', #1664, #14989, #1886, .T. ) ;
#16135=EDGE_LOOP ( 'NONE', ( #36597, #27286 ) ) ;
#16140=VERTEX_POINT ( 'NONE', #10696 ) ;
#16177=PRODUCT ( 'housing left', 'housing left', '', ( #1531 ) ) ;
#16213=DIRECTION ( 'NONE',  ( 1.000000000000000000, 0.000000000000000000, 0.000000000000000000 ) ) ;
#16220=VERTEX_POINT ( 'NONE', #10264 ) ;
#16235=AXIS2_PLACEMENT_3D ( 'NONE', #27307, #40577, #24282 ) ;
#16288=DIRECTION ( 'NONE',  ( 1.000000000000000000, 0.000000000000000000, 0.000000000000000000 ) ) ;
#16448=VERTEX_POINT ( 'NONE', #11281 ) ;
#16493=CIRCLE ( 'NONE', #22091, 2.649999999999985700 ) ;
#16557=ORIENTED_EDGE ( 'NONE', *, *, #21778, .F. ) ;
#16566=ORIENTED_EDGE ( 'NONE', *, *, #33381, .T. ) ;
#16581=CARTESIAN_POINT ( 'NONE',  ( -12.50000000000000000, 1.530808498934191521E-15, -25.00000000000000000 ) ) ;
#16605=CIRCLE ( 'NONE', #9620, 23.00000000000000000 ) ;
#16656=VECTOR ( 'NONE', #18582, 1000.000000000000000 ) ;
#16663=ORIENTED_EDGE ( 'NONE', *, *, #17023, .F. ) ;
#16692=AXIS2_PLACEMENT_3D ( 'NONE', #4387, #17759, #17990 ) ;
#16708=DIRECTION ( 'NONE',  ( 0.000000000000000000, 0.000000000000000000, 1.000000000000000000 ) ) ;
#16731=DIRECTION ( 'NONE',  ( -0.000000000000000000, -0.000000000000000000, -1.000000000000000000 ) ) ;
#16750=EDGE_LOOP ( 'NONE', ( #30579, #38153 ) ) ;
#16761=CARTESIAN_POINT ( 'NONE',  ( 106.4195705685763471, -106.4195705685744855, 6.999999999999998224 ) ) ;
#16787=EDGE_CURVE ( 'NONE', #29580, #3569, #12781, .T. ) ;
#16859=ORIENTED_EDGE ( 'NONE', *, *, #1466, .F. ) ;
#16865=CARTESIAN_POINT ( 'NONE',  ( 0.000000000000000000, 0.000000000000000000, -25.00000000000000000 ) ) ;
#16870=EDGE_CURVE ( 'NONE', #3942, #15086, #20647, .T. ) ;
#16894=EDGE_CURVE ( 'NONE', #21531, #11261, #29013, .T. ) ;
#16917=CARTESIAN_POINT ( 'NONE',  ( -150.5000000000000284, -5.254679414958916394E-13, 9.999999999999998224 ) ) ;
#16936=LINE ( 'NONE', #939, #31752 ) ;
#16960=VERTEX_POINT ( 'NONE', #29861 ) ;
#17023=EDGE_CURVE ( 'NONE', #14989, #1664, #399, .T. ) ;
#17057=ORIENTED_EDGE ( 'NONE', *, *, #40936, .F. ) ;
#17072=DIRECTION ( 'NONE',  ( -0.000000000000000000, -0.000000000000000000, 1.000000000000000000 ) ) ;
#17147=DIRECTION ( 'NONE',  ( 1.000000000000000000, 0.000000000000000000, 0.000000000000000000 ) ) ;
#17149=AXIS2_PLACEMENT_3D ( 'NONE', #1369, #28237, #18233 ) ;
#17159=DIRECTION ( 'NONE',  ( 1.000000000000000000, 0.000000000000000000, 0.000000000000000000 ) ) ;
#17273=DIRECTION ( 'NONE',  ( 0.000000000000000000, 0.000000000000000000, 1.000000000000000000 ) ) ;
#17306=CARTESIAN_POINT ( 'NONE',  ( 0.000000000000000000, 0.000000000000000000, -20.00000000000000000 ) ) ;
#17322=FACE_OUTER_BOUND ( 'NONE', #20527, .T. ) ;
#17333=CARTESIAN_POINT ( 'NONE',  ( 0.000000000000000000, 0.000000000000000000, -25.00000000000000000 ) ) ;
#17369=CARTESIAN_POINT ( 'NONE',  ( 147.8500000000000227, 1.576728355889448963E-12, 6.999999999999998224 ) ) ;
#17483=ORIENTED_EDGE ( 'NONE', *, *, #34108, .F. ) ;
#17500=ORIENTED_EDGE ( 'NONE', *, *, #40201, .F. ) ;
#17511=DIRECTION ( 'NONE',  ( 0.000000000000000000, 0.000000000000000000, 1.000000000000000000 ) ) ;
#17512=DIRECTION ( 'NONE',  ( 0.000000000000000000, 0.000000000000000000, 1.000000000000000000 ) ) ;
#17542=ORIENTED_EDGE ( 'NONE', *, *, #37473, .F. ) ;
#17549=EDGE_CURVE ( 'NONE', #28005, #41293, #6743, .T. ) ;
#17572=DIRECTION ( 'NONE',  ( 0.000000000000000000, 0.000000000000000000, 1.000000000000000000 ) ) ;
#17575=FILL_AREA_STYLE ('',( #10558 ) ) ;
#17590=CARTESIAN_POINT ( 'NONE',  ( 0.000000000000000000, 0.000000000000000000, 6.999999999999998224 ) ) ;
#17627=ORIENTED_EDGE ( 'NONE', *, *, #40540, .F. ) ;
#17637=EDGE_CURVE ( 'NONE', #16220, #23467, #40869, .T. ) ;
#17710=DIRECTION ( 'NONE',  ( 0.000000000000000000, 0.000000000000000000, 1.000000000000000000 ) ) ;
#17715=STYLED_ITEM ( 'NONE', ( #503 ), #3052 ) ;
#17745=DIRECTION ( 'NONE',  ( -0.000000000000000000, -0.000000000000000000, 1.000000000000000000 ) ) ;
#17759=DIRECTION ( 'NONE',  ( 0.000000000000000000, 0.000000000000000000, 1.000000000000000000 ) ) ;
#17809=CARTESIAN_POINT ( 'NONE',  ( -103.7695705685748777, -106.4195705685759776, 10.00000000000000000 ) ) ;
#17851=ADVANCED_FACE ( 'NONE', ( #26677 ), #26252, .T. ) ;
#17879=EDGE_LOOP ( 'NONE', ( #12516, #41285, #27136, #11237 ) ) ;
#17887=ORIENTED_EDGE ( 'NONE', *, *, #31903, .F. ) ;
#17990=DIRECTION ( 'NONE',  ( 1.000000000000000000, 0.000000000000000000, 0.000000000000000000 ) ) ;
#18081=ORIENTED_EDGE ( 'NONE', *, *, #39567, .T. ) ;
#18117=DIRECTION ( 'NONE',  ( 1.000000000000000000, 0.000000000000000000, 0.000000000000000000 ) ) ;
#18134=CARTESIAN_POINT ( 'NONE',  ( -12.50000000000000000, 1.530808498934191521E-15, -20.00000000000000000 ) ) ;
#18188=DIRECTION ( 'NONE',  ( 0.000000000000000000, 0.000000000000000000, 1.000000000000000000 ) ) ;
#18233=DIRECTION ( 'NONE',  ( 1.000000000000000000, 0.000000000000000000, 0.000000000000000000 ) ) ;
#18343=VECTOR ( 'NONE', #42908, 1000.000000000000000 ) ;
#18409=ORIENTED_EDGE ( 'NONE', *, *, #36695, .T. ) ;
#18462=CARTESIAN_POINT ( 'NONE',  ( 0.000000000000000000, 0.000000000000000000, -25.00000000000000000 ) ) ;
#18521=STYLED_ITEM ( 'NONE', ( #19556 ), #27661 ) ;
#18525=ORIENTED_EDGE ( 'NONE', *, *, #40574, .T. ) ;
#18541=EDGE_CURVE ( 'NONE', #28005, #21531, #10681, .T. ) ;
#18542=AXIS2_PLACEMENT_3D ( 'NONE', #3108, #32608, #32813 ) ;
#18576=LINE ( 'NONE', #40990, #943 ) ;
#18582=DIRECTION ( 'NONE',  ( -0.000000000000000000, -0.000000000000000000, 1.000000000000000000 ) ) ;
#18583=AXIS2_PLACEMENT_3D ( 'NONE', #24564, #3767, #17147 ) ;
#18585=AXIS2_PLACEMENT_3D ( 'NONE', #1638, #12136, #5134 ) ;
#18676=CYLINDRICAL_SURFACE ( 'NONE', #7908, 2.649999999999985700 ) ;
#18713=CARTESIAN_POINT ( 'NONE',  ( -2.649999999999993694, -150.5000000000000284, 9.999999999999998224 ) ) ;
#18715=ORIENTED_EDGE ( 'NONE', *, *, #22030, .F. ) ;
#18721=ORIENTED_EDGE ( 'NONE', *, *, #9037, .F. ) ;
#18820=ORIENTED_EDGE ( 'NONE', *, *, #940, .T. ) ;
#18830=DIRECTION ( 'NONE',  ( -0.000000000000000000, -0.000000000000000000, 1.000000000000000000 ) ) ;
#18893=EDGE_CURVE ( 'NONE', #14755, #9269, #2556, .T. ) ;
#18897=DIRECTION ( 'NONE',  ( -0.000000000000000000, -0.000000000000000000, 1.000000000000000000 ) ) ;
#18954=DIRECTION ( 'NONE',  ( 1.000000000000000000, 0.000000000000000000, 0.000000000000000000 ) ) ;
#18961=EDGE_CURVE ( 'NONE', #20768, #34974, #7557, .T. ) ;
#18979=CIRCLE ( 'NONE', #40484, 2.649999999999985700 ) ;
#19021=UNCERTAINTY_MEASURE_WITH_UNIT (LENGTH_MEASURE( 1.000000000000000082E-05 ), #4648, 'distance_accuracy_value', 'NONE');
#19115=FACE_BOUND ( 'NONE', #22713, .T. ) ;
#19158=ORIENTED_EDGE ( 'NONE', *, *, #18961, .T. ) ;
#19231=ORIENTED_EDGE ( 'NONE', *, *, #34366, .T. ) ;
#19311=AXIS2_PLACEMENT_3D ( 'NONE', #32145, #11671, #2226 ) ;
#19335=DIRECTION ( 'NONE',  ( 1.000000000000000000, 0.000000000000000000, 0.000000000000000000 ) ) ;
#19361=ORIENTED_EDGE ( 'NONE', *, *, #41138, .F. ) ;
#19367=CARTESIAN_POINT ( 'NONE',  ( -106.4195705685756081, 106.4195705685752529, 9.999999999999998224 ) ) ;
#19369=FACE_BOUND ( 'NONE', #15720, .T. ) ;
#19377=CARTESIAN_POINT ( 'NONE',  ( -103.7695705685756025, 106.4195705685752529, 9.999999999999998224 ) ) ;
#19398=DIRECTION ( 'NONE',  ( 1.000000000000000000, 0.000000000000000000, 0.000000000000000000 ) ) ;
#19407=AXIS2_PLACEMENT_3D ( 'NONE', #30659, #7728, #21091 ) ;
#19442=EDGE_LOOP ( 'NONE', ( #22626, #31244 ) ) ;
#19457=AXIS2_PLACEMENT_3D ( 'NONE', #2142, #35526, #5644 ) ;
#19488=ORIENTED_EDGE ( 'NONE', *, *, #25003, .F. ) ;
#19545=CARTESIAN_POINT ( 'NONE',  ( -106.4195705685748550, -106.4195705685759776, 6.999999999999998224 ) ) ;
#19553=CARTESIAN_POINT ( 'NONE',  ( -130.0000000000000284, 4.615443851143735910E-16, 367.6955262170047263 ) ) ;
#19556=PRESENTATION_STYLE_ASSIGNMENT (( #2068 ) ) ;
#19576=FACE_BOUND ( 'NONE', #3671, .T. ) ;
#19612=EDGE_CURVE ( 'NONE', #35443, #16220, #8993, .T. ) ;
#19686=AXIS2_PLACEMENT_3D ( 'NONE', #16865, #6785, #24048 ) ;
#19787=VERTEX_POINT ( 'NONE', #19893 ) ;
#19808=DIRECTION ( 'NONE',  ( 1.000000000000000000, 0.000000000000000000, 0.000000000000000000 ) ) ;
#19811=EDGE_CURVE ( 'NONE', #15086, #3942, #42451, .T. ) ;
#19836=CARTESIAN_POINT ( 'NONE',  ( 0.000000000000000000, 150.5000000000000284, 6.999999999999998224 ) ) ;
#19890=LINE ( 'NONE', #9380, #35608 ) ;
#19893=CARTESIAN_POINT ( 'NONE',  ( -20.00000000000000000, 0.000000000000000000, -20.00000000000000000 ) ) ;
#19909=CARTESIAN_POINT ( 'NONE',  ( -106.4195705685748550, -106.4195705685759776, 6.999999999999998224 ) ) ;
#19940=CIRCLE ( 'NONE', #20663, 12.50000000000000000 ) ;
#19969=CARTESIAN_POINT ( 'NONE',  ( 12.50000000000000000, 0.000000000000000000, -25.00000000000000000 ) ) ;
#19976=CARTESIAN_POINT ( 'NONE',  ( 0.000000000000000000, 0.000000000000000000, 6.999999999999998224 ) ) ;
#19992=VECTOR ( 'NONE', #23579, 1000.000000000000000 ) ;
#20054=VERTEX_POINT ( 'NONE', #31207 ) ;
#20067=DIRECTION ( 'NONE',  ( 1.000000000000000000, 0.000000000000000000, 0.000000000000000000 ) ) ;
#20071=ORIENTED_EDGE ( 'NONE', *, *, #39567, .F. ) ;
#20082=DIRECTION ( 'NONE',  ( 1.000000000000000000, 0.000000000000000000, 0.000000000000000000 ) ) ;
#20088=ORIENTED_EDGE ( 'NONE', *, *, #26626, .T. ) ;
#20135=ADVANCED_FACE ( 'NONE', ( #22486 ), #38372, .F. ) ;
#20156=EDGE_LOOP ( 'NONE', ( #5674, #29333, #28270, #15174 ) ) ;
#20158=ADVANCED_FACE ( 'NONE', ( #8490 ), #29016, .F. ) ;
#20172=ORIENTED_EDGE ( 'NONE', *, *, #34298, .F. ) ;
#20207=EDGE_CURVE ( 'NONE', #15962, #20548, #22279, .T. ) ;
#20213=ADVANCED_FACE ( 'NONE', ( #1720 ), #28591, .F. ) ;
#20273=VERTEX_POINT ( 'NONE', #16581 ) ;
#20284=AXIS2_PLACEMENT_3D ( 'NONE', #29459, #42722, #9800 ) ;
#20376=ORIENTED_EDGE ( 'NONE', *, *, #33693, .F. ) ;
#20447=AXIS2_PLACEMENT_3D ( 'NONE', #1891, #15259, #14594 ) ;
#20527=EDGE_LOOP ( 'NONE', ( #10704, #20835, #27838, #31280 ) ) ;
#20542=DIRECTION ( 'NONE',  ( 0.000000000000000000, 0.000000000000000000, 1.000000000000000000 ) ) ;
#20544=CARTESIAN_POINT ( 'NONE',  ( -106.4195705685756081, 106.4195705685752529, 6.999999999999998224 ) ) ;
#20548=VERTEX_POINT ( 'NONE', #24858 ) ;
#20588=MECHANICAL_DESIGN_GEOMETRIC_PRESENTATION_REPRESENTATION('',(#18521),#35185);
#20593=EDGE_LOOP ( 'NONE', ( #24924, #9959, #31617, #16557 ) ) ;
#20629=( LENGTH_UNIT ( ) NAMED_UNIT ( * ) SI_UNIT ( .MILLI., .METRE. ) );
#20647=CIRCLE ( 'NONE', #3166, 130.0000000000000000 ) ;
#20663=AXIS2_PLACEMENT_3D ( 'NONE', #27340, #7471, #24316 ) ;
#20763=CARTESIAN_POINT ( 'NONE',  ( -142.5000000000000284, 1.745121688784978386E-14, 6.999999999999998224 ) ) ;
#20768=VERTEX_POINT ( 'NONE', #23280 ) ;
#20781=ORIENTED_EDGE ( 'NONE', *, *, #19811, .F. ) ;
#20806=CARTESIAN_POINT ( 'NONE',  ( 109.0695705685763244, -106.4195705685744855, 10.00000000000000000 ) ) ;
#20832=ORIENTED_EDGE ( 'NONE', *, *, #29109, .F. ) ;
#20835=ORIENTED_EDGE ( 'NONE', *, *, #444, .F. ) ;
#20900=VECTOR ( 'NONE', #25332, 1000.000000000000000 ) ;
#20940=EDGE_LOOP ( 'NONE', ( #30465, #12273 ) ) ;
#21013=DIRECTION ( 'NONE',  ( 1.000000000000000000, 0.000000000000000000, 0.000000000000000000 ) ) ;
#21029=DIRECTION ( 'NONE',  ( 1.000000000000000000, 0.000000000000000000, 0.000000000000000000 ) ) ;
#21091=DIRECTION ( 'NONE',  ( -1.000000000000000000, 0.000000000000000000, 0.000000000000000000 ) ) ;
#21154=ORIENTED_EDGE ( 'NONE', *, *, #13893, .T. ) ;
#21187=ADVANCED_FACE ( 'NONE', ( #17322 ), #30805, .F. ) ;
#21274=DIRECTION ( 'NONE',  ( 1.000000000000000000, 0.000000000000000000, 0.000000000000000000 ) ) ;
#21293=ORIENTED_EDGE ( 'NONE', *, *, #33430, .F. ) ;
#21314=AXIS2_PLACEMENT_3D ( 'NONE', #22982, #200, #2831 ) ;
#21319=CARTESIAN_POINT ( 'NONE',  ( 0.000000000000000000, -150.5000000000000284, 9.999999999999998224 ) ) ;
#21357=EDGE_CURVE ( 'NONE', #34854, #36509, #4555, .T. ) ;
#21359=LINE ( 'NONE', #8223, #2083 ) ;
#21484=AXIS2_PLACEMENT_3D ( 'NONE', #15600, #11691, #31528 ) ;
#21489=EDGE_LOOP ( 'NONE', ( #25221, #18081, #8830, #16859 ) ) ;
#21510=DIRECTION ( 'NONE',  ( 1.000000000000000000, 0.000000000000000000, -0.000000000000000000 ) ) ;
#21528=CARTESIAN_POINT ( 'NONE',  ( -109.0695705685748607, -106.4195705685759776, 9.999999999999998224 ) ) ;
#21531=VERTEX_POINT ( 'NONE', #15337 ) ;
#21532=FACE_OUTER_BOUND ( 'NONE', #13349, .T. ) ;
#21548=DIRECTION ( 'NONE',  ( 0.000000000000000000, 0.000000000000000000, 1.000000000000000000 ) ) ;
#21558=ADVANCED_FACE ( 'NONE', ( #28629 ), #41902, .F. ) ;
#21589=DIRECTION ( 'NONE',  ( 1.000000000000000000, 0.000000000000000000, 0.000000000000000000 ) ) ;
#21649=DIRECTION ( 'NONE',  ( -1.000000000000000000, 0.000000000000000000, 0.000000000000000000 ) ) ;
#21655=DIRECTION ( 'NONE',  ( 0.000000000000000000, 0.000000000000000000, 1.000000000000000000 ) ) ;
#21670=EDGE_LOOP ( 'NONE', ( #1771, #42140 ) ) ;
#21753=DIRECTION ( 'NONE',  ( 1.000000000000000000, 0.000000000000000000, 0.000000000000000000 ) ) ;
#21778=EDGE_CURVE ( 'NONE', #16960, #36435, #10250, .T. ) ;
#21782=AXIS2_PLACEMENT_3D ( 'NONE', #23175, #33388, #29699 ) ;
#21819=CARTESIAN_POINT ( 'NONE',  ( 103.7695705685741387, 106.4195705685767166, 10.00000000000000000 ) ) ;
#21855=CARTESIAN_POINT ( 'NONE',  ( -150.5000000000000284, -5.254679414958916394E-13, 9.999999999999998224 ) ) ;
#22004=DIRECTION ( 'NONE',  ( 0.000000000000000000, 0.000000000000000000, 1.000000000000000000 ) ) ;
#22030=EDGE_CURVE ( 'NONE', #20054, #14989, #18576, .T. ) ;
#22069=ORIENTED_EDGE ( 'NONE', *, *, #10588, .F. ) ;
#22085=DIRECTION ( 'NONE',  ( 1.000000000000000000, 0.000000000000000000, 0.000000000000000000 ) ) ;
#22091=AXIS2_PLACEMENT_3D ( 'NONE', #16761, #30047, #19808 ) ;
#22105=CARTESIAN_POINT ( 'NONE',  ( 150.5000000000000284, 1.576403824487674918E-12, 9.999999999999998224 ) ) ;
#22117=VERTEX_POINT ( 'NONE', #22275 ) ;
#22130=EDGE_LOOP ( 'NONE', ( #23516, #24043, #42755, #8879 ) ) ;
#22149=DIRECTION ( 'NONE',  ( -0.000000000000000000, -0.000000000000000000, 1.000000000000000000 ) ) ;
#22252=ORIENTED_EDGE ( 'NONE', *, *, #16787, .F. ) ;
#22275=CARTESIAN_POINT ( 'NONE',  ( 142.5000000000000284, 0.000000000000000000, -25.00000000000000000 ) ) ;
#22279=LINE ( 'NONE', #25756, #16656 ) ;
#22310=ORIENTED_EDGE ( 'NONE', *, *, #34108, .T. ) ;
#22323=CIRCLE ( 'NONE', #25797, 126.0000000000000284 ) ;
#22369=DIRECTION ( 'NONE',  ( 1.000000000000000000, 0.000000000000000000, 0.000000000000000000 ) ) ;
#22432=CARTESIAN_POINT ( 'NONE',  ( 0.000000000000000000, 0.000000000000000000, -20.00000000000000000 ) ) ;
#22456=AXIS2_PLACEMENT_3D ( 'NONE', #30199, #37151, #258 ) ;
#22468=EDGE_LOOP ( 'NONE', ( #17542, #27571, #35109, #32712 ) ) ;
#22471=FACE_OUTER_BOUND ( 'NONE', #7531, .T. ) ;
#22473=CIRCLE ( 'NONE', #11301, 2.649999999999985700 ) ;
#22478=AXIS2_PLACEMENT_3D ( 'NONE', #20544, #17710, #40999 ) ;
#22486=FACE_OUTER_BOUND ( 'NONE', #22130, .T. ) ;
#22495=ORIENTED_EDGE ( 'NONE', *, *, #41687, .T. ) ;
#22502=DIRECTION ( 'NONE',  ( 1.000000000000000000, 0.000000000000000000, 0.000000000000000000 ) ) ;
#22547=CARTESIAN_POINT ( 'NONE',  ( -2.649999999999993694, 150.5000000000000284, 9.999999999999998224 ) ) ;
#22598=ADVANCED_FACE ( 'NONE', ( #28543 ), #2505, .F. ) ;
#22621=ORIENTED_EDGE ( 'NONE', *, *, #33981, .F. ) ;
#22626=ORIENTED_EDGE ( 'NONE', *, *, #13717, .F. ) ;
#22710=CARTESIAN_POINT ( 'NONE',  ( 130.0000000000000284, 1.638195277402996435E-14, 367.6955262170047263 ) ) ;
#22713=EDGE_LOOP ( 'NONE', ( #22310, #1292 ) ) ;
#22854=CARTESIAN_POINT ( 'NONE',  ( 5.657435538624008755E-15, 4.615443851143735910E-16, -20.00000000000001776 ) ) ;
#22864=FACE_BOUND ( 'NONE', #24798, .T. ) ;
#22880=ORIENTED_EDGE ( 'NONE', *, *, #34366, .F. ) ;
#22907=ORIENTED_EDGE ( 'NONE', *, *, #8209, .F. ) ;
#22911=CYLINDRICAL_SURFACE ( 'NONE', #27367, 2.649999999999993694 ) ;
#22929=AXIS2_PLACEMENT_3D ( 'NONE', #42285, #12011, #28799 ) ;
#22971=EDGE_CURVE ( 'NONE', #36509, #19787, #31314, .T. ) ;
#22982=CARTESIAN_POINT ( 'NONE',  ( 106.4195705685741302, 106.4195705685767166, 9.999999999999998224 ) ) ;
#23101=DIRECTION ( 'NONE',  ( 0.000000000000000000, 0.000000000000000000, 1.000000000000000000 ) ) ;
#23150=ORIENTED_EDGE ( 'NONE', *, *, #33797, .F. ) ;
#23155=CIRCLE ( 'NONE', #30789, 23.00000000000000000 ) ;
#23175=CARTESIAN_POINT ( 'NONE',  ( 106.4195705685741302, 106.4195705685767166, 10.00000000000000000 ) ) ;
#23179=ORIENTED_EDGE ( 'NONE', *, *, #23420, .F. ) ;
#23278=COLOUR_RGB ( '', 0.09019608, 0.27058824, 0.51372549) ;
#23280=CARTESIAN_POINT ( 'NONE',  ( 2.649999999999993694, 150.5000000000000284, 6.999999999999998224 ) ) ;
#23312=DIRECTION ( 'NONE',  ( 0.000000000000000000, 0.000000000000000000, 1.000000000000000000 ) ) ;
#23349=CIRCLE ( 'NONE', #39294, 2.649999999999999467 ) ;
#23352=VERTEX_POINT ( 'NONE', #4619 ) ;
#23355=DIRECTION ( 'NONE',  ( -0.000000000000000000, -0.000000000000000000, 1.000000000000000000 ) ) ;
#23387=LINE ( 'NONE', #23618, #3447 ) ;
#23401=CARTESIAN_POINT ( 'NONE',  ( 0.000000000000000000, 0.000000000000000000, 9.999999999999998224 ) ) ;
#23420=EDGE_CURVE ( 'NONE', #27122, #30306, #19940, .T. ) ;
#23467=VERTEX_POINT ( 'NONE', #1778 ) ;
#23516=ORIENTED_EDGE ( 'NONE', *, *, #8965, .F. ) ;
#23557=ORIENTED_EDGE ( 'NONE', *, *, #21357, .F. ) ;
#23579=DIRECTION ( 'NONE',  ( -0.000000000000000000, -0.000000000000000000, -1.000000000000000000 ) ) ;
#23618=CARTESIAN_POINT ( 'NONE',  ( 126.0000000000000284, 1.589209405437102375E-14, 367.6955262170047263 ) ) ;
#23672=EDGE_LOOP ( 'NONE', ( #31439, #23931 ) ) ;
#23768=ORIENTED_EDGE ( 'NONE', *, *, #19612, .F. ) ;
#23814=CARTESIAN_POINT ( 'NONE',  ( 139.5000000000000000, 1.708382284810557841E-14, -20.00000000000000000 ) ) ;
#23839=CARTESIAN_POINT ( 'NONE',  ( 0.000000000000000000, 0.000000000000000000, 6.999999999999998224 ) ) ;
#23856=FACE_OUTER_BOUND ( 'NONE', #8533, .T. ) ;
#23913=CARTESIAN_POINT ( 'NONE',  ( 139.5000000000000000, 1.708382284810557841E-14, 9.999999999999998224 ) ) ;
#23931=ORIENTED_EDGE ( 'NONE', *, *, #175, .T. ) ;
#23961=( GEOMETRIC_REPRESENTATION_CONTEXT ( 3 ) GLOBAL_UNCERTAINTY_ASSIGNED_CONTEXT ( ( #19021 ) ) GLOBAL_UNIT_ASSIGNED_CONTEXT ( ( #4648, #1372, #3986 ) ) REPRESENTATION_CONTEXT ( 'NONE', 'WORKASPACE' ) );
#23986=AXIS2_PLACEMENT_3D ( 'NONE', #22105, #31254, #25367 ) ;
#23988=DIRECTION ( 'NONE',  ( 1.000000000000000000, 0.000000000000000000, 0.000000000000000000 ) ) ;
#23998=DIRECTION ( 'NONE',  ( 1.000000000000000000, 0.000000000000000000, 0.000000000000000000 ) ) ;
#24043=ORIENTED_EDGE ( 'NONE', *, *, #7349, .T. ) ;
#24048=DIRECTION ( 'NONE',  ( 1.000000000000000000, 0.000000000000000000, 0.000000000000000000 ) ) ;
#24061=EDGE_CURVE ( 'NONE', #41239, #37517, #25550, .T. ) ;
#24100=AXIS2_PLACEMENT_3D ( 'NONE', #4372, #17745, #21029 ) ;
#24132=LINE ( 'NONE', #23913, #27713 ) ;
#24249=EDGE_CURVE ( 'NONE', #16448, #37680, #8852, .T. ) ;
#24258=FACE_OUTER_BOUND ( 'NONE', #20940, .T. ) ;
#24282=DIRECTION ( 'NONE',  ( 1.000000000000000000, 0.000000000000000000, 0.000000000000000000 ) ) ;
#24316=DIRECTION ( 'NONE',  ( 1.000000000000000000, 0.000000000000000000, 0.000000000000000000 ) ) ;
#24352=CARTESIAN_POINT ( 'NONE',  ( -106.4195705685748550, -106.4195705685759776, 9.999999999999998224 ) ) ;
#24368=EDGE_CURVE ( 'NONE', #3942, #3164, #26174, .T. ) ;
#24401=EDGE_LOOP ( 'NONE', ( #24699, #17887, #28784, #22495 ) ) ;
#24414=CARTESIAN_POINT ( 'NONE',  ( 20.00000000000000000, 2.449293598294706513E-15, -6.000000000000000000 ) ) ;
#24424=CYLINDRICAL_SURFACE ( 'NONE', #20447, 158.5000000000000284 ) ;
#24435=CARTESIAN_POINT ( 'NONE',  ( 0.000000000000000000, 0.000000000000000000, -25.00000000000000000 ) ) ;
#24481=CYLINDRICAL_SURFACE ( 'NONE', #35089, 20.00000000000000000 ) ;
#24534=APPLICATION_CONTEXT ( 'automotive_design' ) ;
#24542=CARTESIAN_POINT ( 'NONE',  ( 0.000000000000000000, 0.000000000000000000, -6.000000000000000000 ) ) ;
#24564=CARTESIAN_POINT ( 'NONE',  ( 0.000000000000000000, 0.000000000000000000, -20.00000000000000000 ) ) ;
#24566=CARTESIAN_POINT ( 'NONE',  ( -158.5000000000000284, 1.941065176648555254E-14, 6.999999999999998224 ) ) ;
#24570=LINE ( 'NONE', #33691, #3294 ) ;
#24598=ORIENTED_EDGE ( 'NONE', *, *, #40936, .T. ) ;
#24699=ORIENTED_EDGE ( 'NONE', *, *, #7349, .F. ) ;
#24752=VERTEX_POINT ( 'NONE', #3276 ) ;
#24774=DIRECTION ( 'NONE',  ( -0.000000000000000000, -0.000000000000000000, 1.000000000000000000 ) ) ;
#24798=EDGE_LOOP ( 'NONE', ( #23150, #13091 ) ) ;
#24808=AXIS2_PLACEMENT_3D ( 'NONE', #23839, #30361, #1270 ) ;
#24858=CARTESIAN_POINT ( 'NONE',  ( -147.8500000000000227, -5.254679414958916394E-13, 10.00000000000000000 ) ) ;
#24866=AXIS2_PLACEMENT_3D ( 'NONE', #38305, #31781, #994 ) ;
#24880=CIRCLE ( 'NONE', #15782, 139.5000000000000000 ) ;
#24922=ADVANCED_FACE ( 'NONE', ( #33831, #3488 ), #6787, .T. ) ;
#24924=ORIENTED_EDGE ( 'NONE', *, *, #35237, .F. ) ;
#24926=DIRECTION ( 'NONE',  ( -0.000000000000000000, -0.000000000000000000, 1.000000000000000000 ) ) ;
#24939=CIRCLE ( 'NONE', #34630, 20.00000000000000000 ) ;
#24973=ORIENTED_EDGE ( 'NONE', *, *, #1595, .T. ) ;
#25003=EDGE_CURVE ( 'NONE', #16220, #35443, #24880, .T. ) ;
#25012=DIRECTION ( 'NONE',  ( 0.000000000000000000, 0.000000000000000000, 1.000000000000000000 ) ) ;
#25177=CARTESIAN_POINT ( 'NONE',  ( 0.000000000000000000, 0.000000000000000000, -25.00000000000000000 ) ) ;
#25204=CIRCLE ( 'NONE', #12652, 2.649999999999993694 ) ;
#25221=ORIENTED_EDGE ( 'NONE', *, *, #40574, .F. ) ;
#25235=FACE_OUTER_BOUND ( 'NONE', #15321, .T. ) ;
#25275=ORIENTED_EDGE ( 'NONE', *, *, #17549, .F. ) ;
#25323=EDGE_LOOP ( 'NONE', ( #20832, #23557 ) ) ;
#25332=DIRECTION ( 'NONE',  ( -0.000000000000000000, -0.000000000000000000, 1.000000000000000000 ) ) ;
#25367=DIRECTION ( 'NONE',  ( 1.000000000000000000, 0.000000000000000000, 0.000000000000000000 ) ) ;
#25401=PRODUCT_DEFINITION_FORMATION_WITH_SPECIFIED_SOURCE ( 'ANY', '', #16177, .NOT_KNOWN. ) ;
#25415=EDGE_LOOP ( 'NONE', ( #10328, #40559, #6507, #28652 ) ) ;
#25443=EDGE_CURVE ( 'NONE', #32065, #3164, #4317, .T. ) ;
#25511=VERTEX_POINT ( 'NONE', #4770 ) ;
#25530=DIRECTION ( 'NONE',  ( 1.000000000000000000, 0.000000000000000000, 0.000000000000000000 ) ) ;
#25543=DIRECTION ( 'NONE',  ( -0.000000000000000000, -0.000000000000000000, 1.000000000000000000 ) ) ;
#25550=CIRCLE ( 'NONE', #42214, 126.0000000000000284 ) ;
#25553=CARTESIAN_POINT ( 'NONE',  ( 0.000000000000000000, 0.000000000000000000, -6.000000000000000000 ) ) ;
#25596=AXIS2_PLACEMENT_3D ( 'NONE', #38105, #8231, #21589 ) ;
#25644=CYLINDRICAL_SURFACE ( 'NONE', #38853, 142.5000000000000284 ) ;
#25756=CARTESIAN_POINT ( 'NONE',  ( -147.8500000000000227, -5.254679414958916394E-13, 9.999999999999998224 ) ) ;
#25797=AXIS2_PLACEMENT_3D ( 'NONE', #22854, #6427, #29373 ) ;
#25804=DIRECTION ( 'NONE',  ( -1.000000000000000000, 0.000000000000000000, 0.000000000000000000 ) ) ;
#25874=LINE ( 'NONE', #15615, #42959 ) ;
#25876=ORIENTED_EDGE ( 'NONE', *, *, #18893, .F. ) ;
#25890=ORIENTED_EDGE ( 'NONE', *, *, #25443, .F. ) ;
#25900=CIRCLE ( 'NONE', #9170, 142.5000000000000284 ) ;
#25905=FACE_BOUND ( 'NONE', #36124, .T. ) ;
#25966=DIRECTION ( 'NONE',  ( 1.000000000000000000, 0.000000000000000000, 0.000000000000000000 ) ) ;
#25975=CIRCLE ( 'NONE', #36403, 2.649999999999985700 ) ;
#25987=DIRECTION ( 'NONE',  ( 1.000000000000000000, 0.000000000000000000, 0.000000000000000000 ) ) ;
#26076=ORIENTED_EDGE ( 'NONE', *, *, #8555, .F. ) ;
#26174=LINE ( 'NONE', #22710, #29050 ) ;
#26202=DIRECTION ( 'NONE',  ( -0.000000000000000000, -0.000000000000000000, 1.000000000000000000 ) ) ;
#26209=EDGE_LOOP ( 'NONE', ( #14554, #3088, #20088, #22252 ) ) ;
#26252=CYLINDRICAL_SURFACE ( 'NONE', #10945, 130.0000000000000284 ) ;
#26296=AXIS2_PLACEMENT_3D ( 'NONE', #29485, #12488, #25804 ) ;
#26308=SURFACE_SIDE_STYLE ('',( #31990 ) ) ;
#26309=CIRCLE ( 'NONE', #11185, 2.649999999999987477 ) ;
#26331=CARTESIAN_POINT ( 'NONE',  ( 109.0695705685741075, 106.4195705685767166, 10.00000000000000000 ) ) ;
#26359=AXIS2_PLACEMENT_3D ( 'NONE', #19836, #33103, #20067 ) ;
#26369=DIRECTION ( 'NONE',  ( -0.000000000000000000, -0.000000000000000000, 1.000000000000000000 ) ) ;
#26395=DIRECTION ( 'NONE',  ( 1.000000000000000000, 0.000000000000000000, 0.000000000000000000 ) ) ;
#26431=DIRECTION ( 'NONE',  ( 0.000000000000000000, 0.000000000000000000, 1.000000000000000000 ) ) ;
#26437=CARTESIAN_POINT ( 'NONE',  ( 0.000000000000000000, 0.000000000000000000, 6.999999999999998224 ) ) ;
#26481=CYLINDRICAL_SURFACE ( 'NONE', #6777, 2.649999999999993694 ) ;
#26626=EDGE_CURVE ( 'NONE', #32160, #3569, #32323, .T. ) ;
#26655=CYLINDRICAL_SURFACE ( 'NONE', #19686, 142.5000000000000284 ) ;
#26677=FACE_OUTER_BOUND ( 'NONE', #36649, .T. ) ;
#26746=CARTESIAN_POINT ( 'NONE',  ( -20.00000000000000000, 0.000000000000000000, -6.000000000000000000 ) ) ;
#26811=DIRECTION ( 'NONE',  ( 0.000000000000000000, 0.000000000000000000, 1.000000000000000000 ) ) ;
#26911=VECTOR ( 'NONE', #9270, 1000.000000000000000 ) ;
#26912=ORIENTED_EDGE ( 'NONE', *, *, #26626, .F. ) ;
#26961=ORIENTED_EDGE ( 'NONE', *, *, #2796, .T. ) ;
#27053=CARTESIAN_POINT ( 'NONE',  ( 23.00000000000000000, 2.816687638038912352E-15, -6.000000000000000000 ) ) ;
#27122=VERTEX_POINT ( 'NONE', #18134 ) ;
#27136=ORIENTED_EDGE ( 'NONE', *, *, #9037, .T. ) ;
#27148=FACE_BOUND ( 'NONE', #7325, .T. ) ;
#27167=ORIENTED_EDGE ( 'NONE', *, *, #41687, .F. ) ;
#27173=FACE_OUTER_BOUND ( 'NONE', #22468, .T. ) ;
#27188=ORIENTED_EDGE ( 'NONE', *, *, #15058, .T. ) ;
#27218=DIRECTION ( 'NONE',  ( 0.000000000000000000, 0.000000000000000000, 1.000000000000000000 ) ) ;
#27286=ORIENTED_EDGE ( 'NONE', *, *, #16894, .T. ) ;
#27293=CARTESIAN_POINT ( 'NONE',  ( 0.000000000000000000, 0.000000000000000000, -6.000000000000000000 ) ) ;
#27307=CARTESIAN_POINT ( 'NONE',  ( -106.4195705685756081, 106.4195705685752529, 10.00000000000000000 ) ) ;
#27339=VECTOR ( 'NONE', #15932, 1000.000000000000000 ) ;
#27340=CARTESIAN_POINT ( 'NONE',  ( 0.000000000000000000, 0.000000000000000000, -20.00000000000000000 ) ) ;
#27346=CIRCLE ( 'NONE', #16235, 2.649999999999985700 ) ;
#27359=DIRECTION ( 'NONE',  ( 1.000000000000000000, 0.000000000000000000, 0.000000000000000000 ) ) ;
#27367=AXIS2_PLACEMENT_3D ( 'NONE', #39844, #26369, #39634 ) ;
#27384=CARTESIAN_POINT ( 'NONE',  ( 0.000000000000000000, -150.5000000000000284, 10.00000000000000000 ) ) ;
#27571=ORIENTED_EDGE ( 'NONE', *, *, #24061, .T. ) ;
#27577=CIRCLE ( 'NONE', #2461, 2.649999999999993694 ) ;
#27582=CARTESIAN_POINT ( 'NONE',  ( 5.657435538624008755E-15, 4.615443851143735910E-16, 367.6955262170047263 ) ) ;
#27590=FACE_OUTER_BOUND ( 'NONE', #20593, .T. ) ;
#27599=VECTOR ( 'NONE', #16708, 1000.000000000000000 ) ;
#27642=CIRCLE ( 'NONE', #19311, 2.649999999999985700 ) ;
#27661=MANIFOLD_SOLID_BREP ( 'CirPattern1', #38594 ) ;
#27687=ORIENTED_EDGE ( 'NONE', *, *, #18961, .F. ) ;
#27713=VECTOR ( 'NONE', #16731, 1000.000000000000000 ) ;
#27719=CARTESIAN_POINT ( 'NONE',  ( -158.5000000000000284, 1.941065176648555254E-14, 6.999999999999998224 ) ) ;
#27744=AXIS2_PLACEMENT_3D ( 'NONE', #14957, #18897, #22369 ) ;
#27790=VERTEX_POINT ( 'NONE', #10786 ) ;
#27813=DIRECTION ( 'NONE',  ( -0.000000000000000000, -0.000000000000000000, -1.000000000000000000 ) ) ;
#27838=ORIENTED_EDGE ( 'NONE', *, *, #8209, .T. ) ;
#27844=DIRECTION ( 'NONE',  ( 1.000000000000000000, 0.000000000000000000, 0.000000000000000000 ) ) ;
#27851=UNCERTAINTY_MEASURE_WITH_UNIT (LENGTH_MEASURE( 1.000000000000000082E-05 ), #39575, 'distance_accuracy_value', 'NONE');
#27888=AXIS2_PLACEMENT_3D ( 'NONE', #19909, #26431, #39701 ) ;
#27931=EDGE_LOOP ( 'NONE', ( #13940, #39006 ) ) ;
#27933=EDGE_CURVE ( 'NONE', #12068, #41700, #16936, .T. ) ;
#27958=DIRECTION ( 'NONE',  ( -1.000000000000000000, 0.000000000000000000, 0.000000000000000000 ) ) ;
#28005=VERTEX_POINT ( 'NONE', #24566 ) ;
#28010=ORIENTED_EDGE ( 'NONE', *, *, #2518, .T. ) ;
#28016=VERTEX_POINT ( 'NONE', #38461 ) ;
#28023=CYLINDRICAL_SURFACE ( 'NONE', #40275, 126.0000000000000284 ) ;
#28045=DIRECTION ( 'NONE',  ( -0.000000000000000000, -0.000000000000000000, -1.000000000000000000 ) ) ;
#28050=EDGE_CURVE ( 'NONE', #5213, #1664, #5317, .T. ) ;
#28113=ADVANCED_FACE ( 'NONE', ( #31723 ), #40870, .F. ) ;
#28237=DIRECTION ( 'NONE',  ( 0.000000000000000000, 0.000000000000000000, 1.000000000000000000 ) ) ;
#28268=VERTEX_POINT ( 'NONE', #30966 ) ;
#28270=ORIENTED_EDGE ( 'NONE', *, *, #33981, .T. ) ;
#28288=EDGE_CURVE ( 'NONE', #24752, #39291, #42178, .T. ) ;
#28344=CIRCLE ( 'NONE', #18583, 139.5000000000000000 ) ;
#28450=VERTEX_POINT ( 'NONE', #20763 ) ;
#28475=ORIENTED_EDGE ( 'NONE', *, *, #28050, .F. ) ;
#28480=ADVANCED_FACE ( 'NONE', ( #31406 ), #42050, .F. ) ;
#28484=ADVANCED_FACE ( 'NONE', ( #11999, #28581 ), #8919, .T. ) ;
#28543=FACE_OUTER_BOUND ( 'NONE', #24401, .T. ) ;
#28581=FACE_OUTER_BOUND ( 'NONE', #9035, .T. ) ;
#28591=CYLINDRICAL_SURFACE ( 'NONE', #19457, 139.5000000000000000 ) ;
#28629=FACE_OUTER_BOUND ( 'NONE', #32359, .T. ) ;
#28652=ORIENTED_EDGE ( 'NONE', *, *, #30164, .F. ) ;
#28748=CARTESIAN_POINT ( 'NONE',  ( 25.26056536696837185, 115.2644951289906885, 0.000000000000000000 ) ) ;
#28784=ORIENTED_EDGE ( 'NONE', *, *, #36479, .T. ) ;
#28799=DIRECTION ( 'NONE',  ( 1.000000000000000000, 0.000000000000000000, 0.000000000000000000 ) ) ;
#28905=CARTESIAN_POINT ( 'NONE',  ( -147.8500000000000227, -5.254679414958916394E-13, 6.999999999999998224 ) ) ;
#28915=FACE_BOUND ( 'NONE', #40657, .T. ) ;
#28937=EDGE_LOOP ( 'NONE', ( #5179, #1439, #7345, #18715 ) ) ;
#28957=CARTESIAN_POINT ( 'NONE',  ( 0.000000000000000000, 0.000000000000000000, 9.999999999999998224 ) ) ;
#28967=EDGE_LOOP ( 'NONE', ( #27167, #37218 ) ) ;
#28979=AXIS2_PLACEMENT_3D ( 'NONE', #4831, #18188, #14891 ) ;
#28984=LINE ( 'NONE', #15280, #10817 ) ;
#29013=CIRCLE ( 'NONE', #7365, 158.5000000000000284 ) ;
#29016=CYLINDRICAL_SURFACE ( 'NONE', #5476, 2.649999999999985700 ) ;
#29050=VECTOR ( 'NONE', #13309, 1000.000000000000000 ) ;
#29051=FACE_OUTER_BOUND ( 'NONE', #31375, .T. ) ;
#29094=CARTESIAN_POINT ( 'NONE',  ( 106.4195705685763471, -106.4195705685744855, 9.999999999999998224 ) ) ;
#29104=ORIENTED_EDGE ( 'NONE', *, *, #29165, .F. ) ;
#29109=EDGE_CURVE ( 'NONE', #36509, #34854, #24939, .T. ) ;
#29127=CARTESIAN_POINT ( 'NONE',  ( 23.00000000000000000, 2.816687638038912352E-15, -20.00000000000000000 ) ) ;
#29142=CARTESIAN_POINT ( 'NONE',  ( -109.0695705685748464, -106.4195705685759776, 10.00000000000000000 ) ) ;
#29165=EDGE_CURVE ( 'NONE', #35443, #30139, #24132, .T. ) ;
#29193=DIRECTION ( 'NONE',  ( 1.000000000000000000, 0.000000000000000000, 0.000000000000000000 ) ) ;
#29218=ORIENTED_EDGE ( 'NONE', *, *, #632, .F. ) ;
#29285=DIRECTION ( 'NONE',  ( 0.000000000000000000, 0.000000000000000000, 1.000000000000000000 ) ) ;
#29333=ORIENTED_EDGE ( 'NONE', *, *, #17549, .T. ) ;
#29355=ADVANCED_FACE ( 'NONE', ( #41961, #1393 ), #11684, .T. ) ;
#29372=CIRCLE ( 'NONE', #35596, 20.00000000000000000 ) ;
#29373=DIRECTION ( 'NONE',  ( 1.000000000000000000, 0.000000000000000000, 0.000000000000000000 ) ) ;
#29425=DIRECTION ( 'NONE',  ( -0.000000000000000000, -0.000000000000000000, -1.000000000000000000 ) ) ;
#29440=CARTESIAN_POINT ( 'NONE',  ( -126.0000000000000284, 4.615443851143735910E-16, 367.6955262170047263 ) ) ;
#29452=PRODUCT_DEFINITION_CONTEXT ( 'detailed design', #15353, 'design' ) ;
#29459=CARTESIAN_POINT ( 'NONE',  ( 5.657435538624008755E-15, 4.615443851143735910E-16, -20.00000000000000000 ) ) ;
#29485=CARTESIAN_POINT ( 'NONE',  ( 0.000000000000000000, 0.000000000000000000, -6.000000000000000000 ) ) ;
#29571=( NAMED_UNIT ( * ) PLANE_ANGLE_UNIT ( ) SI_UNIT ( $, .RADIAN. ) );
#29580=VERTEX_POINT ( 'NONE', #896 ) ;
#29666=CARTESIAN_POINT ( 'NONE',  ( 150.5000000000000284, 1.576403824487674918E-12, 6.999999999999998224 ) ) ;
#29687=DIRECTION ( 'NONE',  ( 0.000000000000000000, 0.000000000000000000, 1.000000000000000000 ) ) ;
#29691=DIRECTION ( 'NONE',  ( -0.000000000000000000, -0.000000000000000000, 1.000000000000000000 ) ) ;
#29699=DIRECTION ( 'NONE',  ( 1.000000000000000000, 0.000000000000000000, 0.000000000000000000 ) ) ;
#29711=CYLINDRICAL_SURFACE ( 'NONE', #21314, 2.649999999999985700 ) ;
#29838=CIRCLE ( 'NONE', #1244, 12.50000000000000000 ) ;
#29861=CARTESIAN_POINT ( 'NONE',  ( 109.0695705685741075, 106.4195705685767166, 6.999999999999998224 ) ) ;
#29898=DIRECTION ( 'NONE',  ( 0.000000000000000000, 0.000000000000000000, 1.000000000000000000 ) ) ;
#29977=ORIENTED_EDGE ( 'NONE', *, *, #18541, .T. ) ;
#29978=DIRECTION ( 'NONE',  ( -0.000000000000000000, -0.000000000000000000, 1.000000000000000000 ) ) ;
#30026=CARTESIAN_POINT ( 'NONE',  ( 106.4195705685741302, 106.4195705685767166, 6.999999999999998224 ) ) ;
#30047=DIRECTION ( 'NONE',  ( 0.000000000000000000, 0.000000000000000000, 1.000000000000000000 ) ) ;
#30127=DIRECTION ( 'NONE',  ( 0.000000000000000000, 0.000000000000000000, 1.000000000000000000 ) ) ;
#30135=CYLINDRICAL_SURFACE ( 'NONE', #26296, 20.00000000000000000 ) ;
#30139=VERTEX_POINT ( 'NONE', #23814 ) ;
#30147=EDGE_CURVE ( 'NONE', #28016, #22117, #31939, .T. ) ;
#30164=EDGE_CURVE ( 'NONE', #10716, #19787, #36694, .T. ) ;
#30177=ORIENTED_EDGE ( 'NONE', *, *, #34904, .T. ) ;
#30183=ORIENTED_EDGE ( 'NONE', *, *, #37504, .F. ) ;
#30199=CARTESIAN_POINT ( 'NONE',  ( 0.000000000000000000, 0.000000000000000000, -6.000000000000000000 ) ) ;
#30224=ORIENTED_EDGE ( 'NONE', *, *, #30757, .F. ) ;
#30250=ADVANCED_FACE ( 'NONE', ( #847, #24258 ), #32009, .T. ) ;
#30269=CARTESIAN_POINT ( 'NONE',  ( -4.943662031389838196E-16, -1.828353205453026285E-14, 6.938893903907228378E-15 ) ) ;
#30306=VERTEX_POINT ( 'NONE', #33288 ) ;
#30349=CARTESIAN_POINT ( 'NONE',  ( -126.0000000000000284, 4.615443851143735910E-16, 0.000000000000000000 ) ) ;
#30361=DIRECTION ( 'NONE',  ( 0.000000000000000000, 0.000000000000000000, 1.000000000000000000 ) ) ;
#30419=DIRECTION ( 'NONE',  ( -0.000000000000000000, -0.000000000000000000, 1.000000000000000000 ) ) ;
#30462=AXIS2_PLACEMENT_3D ( 'NONE', #17590, #25012, #38255 ) ;
#30465=ORIENTED_EDGE ( 'NONE', *, *, #19811, .T. ) ;
#30505=CIRCLE ( 'NONE', #21484, 2.649999999999987477 ) ;
#30575=EDGE_LOOP ( 'NONE', ( #14081, #25275 ) ) ;
#30579=ORIENTED_EDGE ( 'NONE', *, *, #31903, .T. ) ;
#30634=ORIENTED_EDGE ( 'NONE', *, *, #12072, .F. ) ;
#30659=CARTESIAN_POINT ( 'NONE',  ( 5.657435538624008755E-15, 4.615443851143735910E-16, 367.6955262170047263 ) ) ;
#30757=EDGE_CURVE ( 'NONE', #23352, #38293, #30505, .T. ) ;
#30759=CIRCLE ( 'NONE', #2172, 23.00000000000000000 ) ;
#30766=CARTESIAN_POINT ( 'NONE',  ( 109.0695705685741075, 106.4195705685767166, 9.999999999999998224 ) ) ;
#30789=AXIS2_PLACEMENT_3D ( 'NONE', #24542, #7914, #21274 ) ;
#30792=ADVANCED_FACE ( 'NONE', ( #37831 ), #41544, .F. ) ;
#30805=CYLINDRICAL_SURFACE ( 'NONE', #24100, 2.649999999999985700 ) ;
#30830=ADVANCED_FACE ( 'NONE', ( #9242 ), #26481, .F. ) ;
#30966=CARTESIAN_POINT ( 'NONE',  ( 142.5000000000000284, 0.000000000000000000, 6.999999999999998224 ) ) ;
#31094=CARTESIAN_POINT ( 'NONE',  ( -20.00000000000000000, 0.000000000000000000, -6.000000000000000000 ) ) ;
#31111=CARTESIAN_POINT ( 'NONE',  ( 2.649999999999993694, -150.5000000000000284, 9.999999999999998224 ) ) ;
#31116=AXIS2_PLACEMENT_3D ( 'NONE', #15894, #33074, #29193 ) ;
#31149=ORIENTED_EDGE ( 'NONE', *, *, #16870, .F. ) ;
#31183=AXIS2_PLACEMENT_3D ( 'NONE', #30026, #13882, #1394 ) ;
#31196=DIRECTION ( 'NONE',  ( 1.000000000000000000, 0.000000000000000000, 0.000000000000000000 ) ) ;
#31207=CARTESIAN_POINT ( 'NONE',  ( -103.7695705685748635, -106.4195705685759776, 6.999999999999998224 ) ) ;
#31226=ADVANCED_FACE ( 'NONE', ( #11150 ), #24481, .F. ) ;
#31244=ORIENTED_EDGE ( 'NONE', *, *, #41786, .F. ) ;
#31254=DIRECTION ( 'NONE',  ( -0.000000000000000000, -0.000000000000000000, 1.000000000000000000 ) ) ;
#31261=ORIENTED_EDGE ( 'NONE', *, *, #25443, .T. ) ;
#31280=ORIENTED_EDGE ( 'NONE', *, *, #33797, .T. ) ;
#31295=ORIENTED_EDGE ( 'NONE', *, *, #1466, .T. ) ;
#31301=CIRCLE ( 'NONE', #40327, 2.649999999999985700 ) ;
#31307=DIRECTION ( 'NONE',  ( 1.000000000000000000, 0.000000000000000000, 0.000000000000000000 ) ) ;
#31310=ADVANCED_FACE ( 'NONE', ( #9141 ), #38383, .T. ) ;
#31314=LINE ( 'NONE', #31094, #9431 ) ;
#31321=ORIENTED_EDGE ( 'NONE', *, *, #940, .F. ) ;
#31375=EDGE_LOOP ( 'NONE', ( #31811, #33543, #12268, #18820 ) ) ;
#31406=FACE_OUTER_BOUND ( 'NONE', #40408, .T. ) ;
#31439=ORIENTED_EDGE ( 'NONE', *, *, #33693, .T. ) ;
#31528=DIRECTION ( 'NONE',  ( 1.000000000000000000, 0.000000000000000000, 0.000000000000000000 ) ) ;
#31617=ORIENTED_EDGE ( 'NONE', *, *, #8796, .T. ) ;
#31626=EDGE_CURVE ( 'NONE', #5016, #27790, #5893, .T. ) ;
#31702=VECTOR ( 'NONE', #32541, 1000.000000000000000 ) ;
#31723=FACE_OUTER_BOUND ( 'NONE', #4187, .T. ) ;
#31732=CIRCLE ( 'NONE', #18542, 2.649999999999985700 ) ;
#31752=VECTOR ( 'NONE', #39790, 1000.000000000000000 ) ;
#31781=DIRECTION ( 'NONE',  ( -0.000000000000000000, -0.000000000000000000, 1.000000000000000000 ) ) ;
#31811=ORIENTED_EDGE ( 'NONE', *, *, #40550, .F. ) ;
#31839=EDGE_LOOP ( 'NONE', ( #30634, #17483, #14602, #24598 ) ) ;
#31903=EDGE_CURVE ( 'NONE', #25511, #2475, #23349, .T. ) ;
#31939=CIRCLE ( 'NONE', #13134, 142.5000000000000284 ) ;
#31951=FACE_OUTER_BOUND ( 'NONE', #28937, .T. ) ;
#31990=SURFACE_STYLE_FILL_AREA ( #13005 ) ;
#32009=PLANE ( 'NONE',  #40177 ) ;
#32060=CARTESIAN_POINT ( 'NONE',  ( 142.5000000000000284, 0.000000000000000000, -25.00000000000000000 ) ) ;
#32065=VERTEX_POINT ( 'NONE', #312 ) ;
#32145=CARTESIAN_POINT ( 'NONE',  ( 150.5000000000000284, 1.576403824487674918E-12, 10.00000000000000000 ) ) ;
#32160=VERTEX_POINT ( 'NONE', #14491 ) ;
#32172=FACE_BOUND ( 'NONE', #875, .T. ) ;
#32323=CIRCLE ( 'NONE', #42053, 2.649999999999985700 ) ;
#32347=CIRCLE ( 'NONE', #12166, 2.649999999999985700 ) ;
#32359=EDGE_LOOP ( 'NONE', ( #8551, #12426, #21154, #22907 ) ) ;
#32496=CARTESIAN_POINT ( 'NONE',  ( -2.649999999999993694, -150.5000000000000284, 6.999999999999998224 ) ) ;
#32531=CARTESIAN_POINT ( 'NONE',  ( -106.4195705685748550, -106.4195705685759776, 10.00000000000000000 ) ) ;
#32541=DIRECTION ( 'NONE',  ( -0.000000000000000000, -0.000000000000000000, 1.000000000000000000 ) ) ;
#32577=EDGE_LOOP ( 'NONE', ( #25890, #40649 ) ) ;
#32608=DIRECTION ( 'NONE',  ( -0.000000000000000000, -0.000000000000000000, 1.000000000000000000 ) ) ;
#32695=CARTESIAN_POINT ( 'NONE',  ( -23.00000000000000000, 0.000000000000000000, -20.00000000000000000 ) ) ;
#32712=ORIENTED_EDGE ( 'NONE', *, *, #12100, .T. ) ;
#32718=CARTESIAN_POINT ( 'NONE',  ( 130.0000000000000000, 1.638195277402996435E-14, 6.938893903907228378E-15 ) ) ;
#32749=DIRECTION ( 'NONE',  ( 1.000000000000000000, 0.000000000000000000, 0.000000000000000000 ) ) ;
#32805=VECTOR ( 'NONE', #14361, 1000.000000000000000 ) ;
#32813=DIRECTION ( 'NONE',  ( 1.000000000000000000, 0.000000000000000000, 0.000000000000000000 ) ) ;
#32930=AXIS2_PLACEMENT_3D ( 'NONE', #41396, #35077, #8469 ) ;
#33074=DIRECTION ( 'NONE',  ( 0.000000000000000000, 0.000000000000000000, 1.000000000000000000 ) ) ;
#33086=CIRCLE ( 'NONE', #38655, 142.5000000000000284 ) ;
#33093=DIRECTION ( 'NONE',  ( -0.2140725878556641593, -0.9768177553304296934, 0.000000000000000000 ) ) ;
#33103=DIRECTION ( 'NONE',  ( 0.000000000000000000, 0.000000000000000000, 1.000000000000000000 ) ) ;
#33116=CIRCLE ( 'NONE', #12247, 142.5000000000000284 ) ;
#33132=CARTESIAN_POINT ( 'NONE',  ( -150.5000000000000284, -5.254679414958916394E-13, 6.999999999999998224 ) ) ;
#33205=ORIENTED_EDGE ( 'NONE', *, *, #41138, .T. ) ;
#33227=ORIENTED_EDGE ( 'NONE', *, *, #8374, .F. ) ;
#33288=CARTESIAN_POINT ( 'NONE',  ( 12.50000000000000000, 0.000000000000000000, -20.00000000000000000 ) ) ;
#33381=EDGE_CURVE ( 'NONE', #2582, #29580, #16493, .T. ) ;
#33388=DIRECTION ( 'NONE',  ( -0.000000000000000000, -0.000000000000000000, 1.000000000000000000 ) ) ;
#33430=EDGE_CURVE ( 'NONE', #20273, #36979, #15801, .T. ) ;
#33543=ORIENTED_EDGE ( 'NONE', *, *, #15812, .F. ) ;
#33670=ORIENTED_EDGE ( 'NONE', *, *, #29109, .T. ) ;
#33691=CARTESIAN_POINT ( 'NONE',  ( 20.00000000000000000, 2.449293598294706513E-15, -6.000000000000000000 ) ) ;
#33693=EDGE_CURVE ( 'NONE', #28268, #28450, #33116, .T. ) ;
#33738=CARTESIAN_POINT ( 'NONE',  ( 0.000000000000000000, 0.000000000000000000, 9.999999999999998224 ) ) ;
#33782=CARTESIAN_POINT ( 'NONE',  ( 5.657435538624008755E-15, 4.615443851143735910E-16, -20.00000000000000000 ) ) ;
#33784=EDGE_CURVE ( 'NONE', #5213, #20054, #40071, .T. ) ;
#33785=CARTESIAN_POINT ( 'NONE',  ( 103.7695705685763556, -106.4195705685744855, 9.999999999999998224 ) ) ;
#33797=EDGE_CURVE ( 'NONE', #16140, #39372, #31732, .T. ) ;
#33800=EDGE_CURVE ( 'NONE', #36979, #30306, #9476, .T. ) ;
#33831=FACE_BOUND ( 'NONE', #32577, .T. ) ;
#33981=EDGE_CURVE ( 'NONE', #41293, #11261, #7706, .T. ) ;
#34007=CIRCLE ( 'NONE', #1951, 2.649999999999987477 ) ;
#34102=FACE_OUTER_BOUND ( 'NONE', #30575, .T. ) ;
#34108=EDGE_CURVE ( 'NONE', #16960, #8432, #11561, .T. ) ;
#34196=CARTESIAN_POINT ( 'NONE',  ( -150.5000000000000284, -5.254679414958916394E-13, 6.999999999999998224 ) ) ;
#34211=CARTESIAN_POINT ( 'NONE',  ( 106.4195705685741302, 106.4195705685767166, 10.00000000000000000 ) ) ;
#34298=EDGE_CURVE ( 'NONE', #2582, #32160, #3225, .T. ) ;
#34340=CARTESIAN_POINT ( 'NONE',  ( -130.0000000000000000, 4.615443851143692522E-16, 6.938893903907228378E-15 ) ) ;
#34343=CARTESIAN_POINT ( 'NONE',  ( 0.000000000000000000, 0.000000000000000000, -6.000000000000000000 ) ) ;
#34364=ORIENTED_EDGE ( 'NONE', *, *, #33784, .T. ) ;
#34366=EDGE_CURVE ( 'NONE', #7826, #36784, #13527, .T. ) ;
#34421=DIRECTION ( 'NONE',  ( 1.000000000000000000, 0.000000000000000000, 0.000000000000000000 ) ) ;
#34459=ORIENTED_EDGE ( 'NONE', *, *, #17023, .T. ) ;
#34528=CIRCLE ( 'NONE', #3821, 2.649999999999985700 ) ;
#34573=EDGE_LOOP ( 'NONE', ( #7694, #22069 ) ) ;
#34629=FACE_OUTER_BOUND ( 'NONE', #20156, .T. ) ;
#34630=AXIS2_PLACEMENT_3D ( 'NONE', #34343, #7288, #17159 ) ;
#34635=CARTESIAN_POINT ( 'NONE',  ( -106.4195705685756081, 106.4195705685752529, 6.999999999999998224 ) ) ;
#34740=DIRECTION ( 'NONE',  ( 0.000000000000000000, 0.000000000000000000, 1.000000000000000000 ) ) ;
#34777=CIRCLE ( 'NONE', #2695, 2.649999999999993694 ) ;
#34828=DIRECTION ( 'NONE',  ( -0.000000000000000000, -0.000000000000000000, 1.000000000000000000 ) ) ;
#34854=VERTEX_POINT ( 'NONE', #24414 ) ;
#34904=EDGE_CURVE ( 'NONE', #3569, #32160, #35969, .T. ) ;
#34929=AXIS2_PLACEMENT_3D ( 'NONE', #28957, #22004, #12163 ) ;
#34971=ORIENTED_EDGE ( 'NONE', *, *, #42992, .T. ) ;
#34974=VERTEX_POINT ( 'NONE', #9509 ) ;
#35077=DIRECTION ( 'NONE',  ( -0.000000000000000000, -0.000000000000000000, -1.000000000000000000 ) ) ;
#35089=AXIS2_PLACEMENT_3D ( 'NONE', #27293, #10699, #27958 ) ;
#35091=CARTESIAN_POINT ( 'NONE',  ( 106.4195705685763471, -106.4195705685744855, 9.999999999999998224 ) ) ;
#35103=DIRECTION ( 'NONE',  ( 0.000000000000000000, 0.000000000000000000, 1.000000000000000000 ) ) ;
#35104=LINE ( 'NONE', #19377, #20900 ) ;
#35109=ORIENTED_EDGE ( 'NONE', *, *, #9272, .T. ) ;
#35146=AXIS2_PLACEMENT_3D ( 'NONE', #33132, #26811, #43154 ) ;
#35185=( GEOMETRIC_REPRESENTATION_CONTEXT ( 3 ) GLOBAL_UNCERTAINTY_ASSIGNED_CONTEXT ( ( #27851 ) ) GLOBAL_UNIT_ASSIGNED_CONTEXT ( ( #39575, #29571, #35868 ) ) REPRESENTATION_CONTEXT ( 'NONE', 'WORKASPACE' ) );
#35200=DIRECTION ( 'NONE',  ( 1.000000000000000000, 0.000000000000000000, 0.000000000000000000 ) ) ;
#35214=EDGE_LOOP ( 'NONE', ( #33205, #38629 ) ) ;
#35237=EDGE_CURVE ( 'NONE', #8432, #16960, #3945, .T. ) ;
#35283=AXIS2_PLACEMENT_3D ( 'NONE', #38564, #4995, #12427 ) ;
#35339=DIRECTION ( 'NONE',  ( 0.000000000000000000, 0.000000000000000000, 1.000000000000000000 ) ) ;
#35420=ORIENTED_EDGE ( 'NONE', *, *, #24061, .F. ) ;
#35422=ORIENTED_EDGE ( 'NONE', *, *, #30757, .T. ) ;
#35443=VERTEX_POINT ( 'NONE', #15595 ) ;
#35446=DIRECTION ( 'NONE',  ( 0.000000000000000000, 0.000000000000000000, 1.000000000000000000 ) ) ;
#35526=DIRECTION ( 'NONE',  ( -0.000000000000000000, -0.000000000000000000, -1.000000000000000000 ) ) ;
#35549=CYLINDRICAL_SURFACE ( 'NONE', #11371, 2.649999999999993694 ) ;
#35596=AXIS2_PLACEMENT_3D ( 'NONE', #6654, #3782, #80 ) ;
#35608=VECTOR ( 'NONE', #29691, 1000.000000000000000 ) ;
#35620=CARTESIAN_POINT ( 'NONE',  ( 5.657435538624008755E-15, 4.615443851143735910E-16, 367.6955262170047263 ) ) ;
#35681=FACE_BOUND ( 'NONE', #27931, .T. ) ;
#35687=CARTESIAN_POINT ( 'NONE',  ( -126.0000000000000284, 4.615443851143735910E-16, -20.00000000000001776 ) ) ;
#35746=FACE_OUTER_BOUND ( 'NONE', #21489, .T. ) ;
#35774=DIRECTION ( 'NONE',  ( -0.000000000000000000, -0.000000000000000000, 1.000000000000000000 ) ) ;
#35852=PRODUCT_DEFINITION ( 'UNKNOWN', '', #25401, #29452 ) ;
#35868=( NAMED_UNIT ( * ) SI_UNIT ( $, .STERADIAN. ) SOLID_ANGLE_UNIT ( ) );
#35921=AXIS2_PLACEMENT_3D ( 'NONE', #24352, #37606, #7724 ) ;
#35969=CIRCLE ( 'NONE', #25596, 2.649999999999985700 ) ;
#35987=CYLINDRICAL_SURFACE ( 'NONE', #7434, 12.50000000000000000 ) ;
#36115=FACE_BOUND ( 'NONE', #7412, .T. ) ;
#36124=EDGE_LOOP ( 'NONE', ( #8565, #26912 ) ) ;
#36171=LINE ( 'NONE', #29440, #27339 ) ;
#36190=DIRECTION ( 'NONE',  ( -0.000000000000000000, -0.000000000000000000, 1.000000000000000000 ) ) ;
#36309=AXIS2_PLACEMENT_3D ( 'NONE', #2926, #39373, #16288 ) ;
#36403=AXIS2_PLACEMENT_3D ( 'NONE', #34196, #362, #20082 ) ;
#36435=VERTEX_POINT ( 'NONE', #26331 ) ;
#36479=EDGE_CURVE ( 'NONE', #25511, #27790, #35104, .T. ) ;
#36509=VERTEX_POINT ( 'NONE', #26746 ) ;
#36534=DIRECTION ( 'NONE',  ( 1.000000000000000000, 0.000000000000000000, 0.000000000000000000 ) ) ;
#36590=EDGE_CURVE ( 'NONE', #29580, #2582, #31301, .T. ) ;
#36597=ORIENTED_EDGE ( 'NONE', *, *, #40540, .T. ) ;
#36600=ORIENTED_EDGE ( 'NONE', *, *, #8796, .F. ) ;
#36635=DIRECTION ( 'NONE',  ( -0.000000000000000000, -0.000000000000000000, 1.000000000000000000 ) ) ;
#36649=EDGE_LOOP ( 'NONE', ( #42115, #20781, #34971, #31261 ) ) ;
#36676=AXIS2_PLACEMENT_3D ( 'NONE', #14727, #24774, #14510 ) ;
#36687=VECTOR ( 'NONE', #7723, 1000.000000000000000 ) ;
#36694=CIRCLE ( 'NONE', #9561, 20.00000000000000000 ) ;
#36695=EDGE_CURVE ( 'NONE', #34974, #20768, #34777, .T. ) ;
#36722=FACE_OUTER_BOUND ( 'NONE', #6057, .T. ) ;
#36733=ADVANCED_FACE ( 'NONE', ( #25235 ), #11467, .F. ) ;
#36784=VERTEX_POINT ( 'NONE', #29127 ) ;
#36889=CARTESIAN_POINT ( 'NONE',  ( -153.1500000000000057, -5.251434100941175950E-13, 10.00000000000000000 ) ) ;
#36892=ORIENTED_EDGE ( 'NONE', *, *, #17637, .T. ) ;
#36979=VERTEX_POINT ( 'NONE', #19969 ) ;
#36988=CARTESIAN_POINT ( 'NONE',  ( 158.5000000000000284, 0.000000000000000000, 9.999999999999998224 ) ) ;
#37020=ORIENTED_EDGE ( 'NONE', *, *, #13430, .T. ) ;
#37022=ORIENTED_EDGE ( 'NONE', *, *, #15054, .T. ) ;
#37042=DIRECTION ( 'NONE',  ( -0.000000000000000000, -0.000000000000000000, 1.000000000000000000 ) ) ;
#37080=CARTESIAN_POINT ( 'NONE',  ( -4.943662031389838196E-16, -1.828353205453026285E-14, 6.938893903907228378E-15 ) ) ;
#37151=DIRECTION ( 'NONE',  ( 0.000000000000000000, 0.000000000000000000, 1.000000000000000000 ) ) ;
#37156=( GEOMETRIC_REPRESENTATION_CONTEXT ( 3 ) GLOBAL_UNCERTAINTY_ASSIGNED_CONTEXT ( ( #15949 ) ) GLOBAL_UNIT_ASSIGNED_CONTEXT ( ( #20629, #7709, #711 ) ) REPRESENTATION_CONTEXT ( 'NONE', 'WORKASPACE' ) );
#37218=ORIENTED_EDGE ( 'NONE', *, *, #31626, .F. ) ;
#37286=ORIENTED_EDGE ( 'NONE', *, *, #12100, .F. ) ;
#37292=EDGE_LOOP ( 'NONE', ( #28010, #18525 ) ) ;
#37371=DIRECTION ( 'NONE',  ( 1.000000000000000000, 0.000000000000000000, -0.000000000000000000 ) ) ;
#37473=EDGE_CURVE ( 'NONE', #41239, #24752, #23387, .T. ) ;
#37504=EDGE_CURVE ( 'NONE', #20054, #5213, #2084, .T. ) ;
#37517=VERTEX_POINT ( 'NONE', #30349 ) ;
#37565=ORIENTED_EDGE ( 'NONE', *, *, #14997, .T. ) ;
#37593=SURFACE_STYLE_FILL_AREA ( #17575 ) ;
#37605=CARTESIAN_POINT ( 'NONE',  ( -139.5000000000000000, 0.000000000000000000, 9.999999999999998224 ) ) ;
#37606=DIRECTION ( 'NONE',  ( -0.000000000000000000, -0.000000000000000000, 1.000000000000000000 ) ) ;
#37680=VERTEX_POINT ( 'NONE', #7425 ) ;
#37747=DIRECTION ( 'NONE',  ( 1.000000000000000000, 0.000000000000000000, 0.000000000000000000 ) ) ;
#37822=DIRECTION ( 'NONE',  ( 1.000000000000000000, 0.000000000000000000, 0.000000000000000000 ) ) ;
#37825=CARTESIAN_POINT ( 'NONE',  ( 0.000000000000000000, 0.000000000000000000, -6.000000000000000000 ) ) ;
#37831=FACE_OUTER_BOUND ( 'NONE', #7016, .T. ) ;
#37877=CARTESIAN_POINT ( 'NONE',  ( -150.5000000000000284, -5.254679414958916394E-13, 10.00000000000000000 ) ) ;
#37905=DIRECTION ( 'NONE',  ( -0.000000000000000000, -0.000000000000000000, 1.000000000000000000 ) ) ;
#37911=CYLINDRICAL_SURFACE ( 'NONE', #24808, 158.5000000000000284 ) ;
#38018=AXIS2_PLACEMENT_3D ( 'NONE', #1052, #40757, #31196 ) ;
#38105=CARTESIAN_POINT ( 'NONE',  ( 106.4195705685763471, -106.4195705685744855, 10.00000000000000000 ) ) ;
#38137=DIRECTION ( 'NONE',  ( -0.000000000000000000, -0.000000000000000000, 1.000000000000000000 ) ) ;
#38141=FACE_OUTER_BOUND ( 'NONE', #41759, .T. ) ;
#38153=ORIENTED_EDGE ( 'NONE', *, *, #8965, .T. ) ;
#38176=DIRECTION ( 'NONE',  ( -0.000000000000000000, -0.000000000000000000, -1.000000000000000000 ) ) ;
#38255=DIRECTION ( 'NONE',  ( 1.000000000000000000, 0.000000000000000000, 0.000000000000000000 ) ) ;
#38293=VERTEX_POINT ( 'NONE', #38334 ) ;
#38305=CARTESIAN_POINT ( 'NONE',  ( -106.4195705685748550, -106.4195705685759776, 10.00000000000000000 ) ) ;
#38324=VERTEX_POINT ( 'NONE', #21819 ) ;
#38334=CARTESIAN_POINT ( 'NONE',  ( 2.649999999999987477, 150.5000000000000284, 10.00000000000000000 ) ) ;
#38372=CYLINDRICAL_SURFACE ( 'NONE', #22929, 2.649999999999999467 ) ;
#38383=CYLINDRICAL_SURFACE ( 'NONE', #12836, 23.00000000000000000 ) ;
#38393=DIRECTION ( 'NONE',  ( 1.000000000000000000, 0.000000000000000000, -0.000000000000000000 ) ) ;
#38461=CARTESIAN_POINT ( 'NONE',  ( -142.5000000000000284, 1.745121688784978386E-14, -25.00000000000000000 ) ) ;
#38467=CYLINDRICAL_SURFACE ( 'NONE', #27744, 2.649999999999999467 ) ;
#38475=ORIENTED_EDGE ( 'NONE', *, *, #29165, .T. ) ;
#38491=DIRECTION ( 'NONE',  ( -0.000000000000000000, -0.000000000000000000, 1.000000000000000000 ) ) ;
#38564=CARTESIAN_POINT ( 'NONE',  ( 0.000000000000000000, 0.000000000000000000, -20.00000000000000000 ) ) ;
#38594=CLOSED_SHELL ( 'NONE', ( #6720, #21558, #6910, #41995, #15191, #20158, #20135, #30830, #2189, #36733, #5493, #15229, #16060, #31310, #11614, #40253, #15207, #24922, #40350, #28484, #5468, #14387, #29355, #42261, #31226, #17851, #15134, #30250, #8307, #20213, #9670, #39711, #11737, #22598, #41230, #28113, #30792, #28480, #21187, #161 ) ) ;
#38615=ORIENTED_EDGE ( 'NONE', *, *, #42992, .F. ) ;
#38629=ORIENTED_EDGE ( 'NONE', *, *, #40006, .T. ) ;
#38655=AXIS2_PLACEMENT_3D ( 'NONE', #26437, #29285, #32749 ) ;
#38725=FILL_AREA_STYLE_COLOUR ( '', #15694 ) ;
#38853=AXIS2_PLACEMENT_3D ( 'NONE', #18462, #12318, #35200 ) ;
#38902=DIRECTION ( 'NONE',  ( -1.000000000000000000, 0.000000000000000000, 0.000000000000000000 ) ) ;
#38922=FACE_BOUND ( 'NONE', #41626, .T. ) ;
#38957=FACE_BOUND ( 'NONE', #28967, .T. ) ;
#39006=ORIENTED_EDGE ( 'NONE', *, *, #24249, .F. ) ;
#39038=CIRCLE ( 'NONE', #20284, 130.0000000000000284 ) ;
#39051=DIRECTION ( 'NONE',  ( 1.000000000000000000, 0.000000000000000000, 0.000000000000000000 ) ) ;
#39076=VECTOR ( 'NONE', #5345, 1000.000000000000000 ) ;
#39082=SHAPE_REPRESENTATION ( 'housing left', ( #13552 ), #23961 ) ;
#39137=CARTESIAN_POINT ( 'NONE',  ( -109.0695705685748607, -106.4195705685759776, 6.999999999999998224 ) ) ;
#39149=CARTESIAN_POINT ( 'NONE',  ( 109.0695705685763244, -106.4195705685744855, 9.999999999999998224 ) ) ;
#39291=VERTEX_POINT ( 'NONE', #35687 ) ;
#39294=AXIS2_PLACEMENT_3D ( 'NONE', #34635, #1678, #18117 ) ;
#39299=EDGE_LOOP ( 'NONE', ( #11487, #24973, #20376, #18721 ) ) ;
#39372=VERTEX_POINT ( 'NONE', #7538 ) ;
#39373=DIRECTION ( 'NONE',  ( 0.000000000000000000, 0.000000000000000000, 1.000000000000000000 ) ) ;
#39555=ORIENTED_EDGE ( 'NONE', *, *, #15812, .T. ) ;
#39567=EDGE_CURVE ( 'NONE', #40561, #16448, #5119, .T. ) ;
#39575=( LENGTH_UNIT ( ) NAMED_UNIT ( * ) SI_UNIT ( .MILLI., .METRE. ) );
#39634=DIRECTION ( 'NONE',  ( 1.000000000000000000, 0.000000000000000000, 0.000000000000000000 ) ) ;
#39639=AXIS2_PLACEMENT_3D ( 'NONE', #41765, #8184, #7745 ) ;
#39701=DIRECTION ( 'NONE',  ( 1.000000000000000000, 0.000000000000000000, 0.000000000000000000 ) ) ;
#39711=ADVANCED_FACE ( 'NONE', ( #19115, #32172, #28915, #12340, #38922, #9039, #15827, #27148, #40618, #34102 ), #14061, .F. ) ;
#39777=CARTESIAN_POINT ( 'NONE',  ( 2.649999999999993694, -150.5000000000000284, 6.999999999999998224 ) ) ;
#39790=DIRECTION ( 'NONE',  ( -0.000000000000000000, -0.000000000000000000, 1.000000000000000000 ) ) ;
#39827=AXIS2_PLACEMENT_3D ( 'NONE', #16917, #30419, #27359 ) ;
#39829=CARTESIAN_POINT ( 'NONE',  ( 0.000000000000000000, -150.5000000000000284, 6.999999999999998224 ) ) ;
#39844=CARTESIAN_POINT ( 'NONE',  ( 0.000000000000000000, 150.5000000000000284, 9.999999999999998224 ) ) ;
#39910=ORIENTED_EDGE ( 'NONE', *, *, #33800, .F. ) ;
#39930=VECTOR ( 'NONE', #36635, 1000.000000000000000 ) ;
#40006=EDGE_CURVE ( 'NONE', #7826, #14755, #23155, .T. ) ;
#40043=EDGE_LOOP ( 'NONE', ( #33227, #35420 ) ) ;
#40071=CIRCLE ( 'NONE', #7324, 2.649999999999999467 ) ;
#40147=DIRECTION ( 'NONE',  ( 1.000000000000000000, 0.000000000000000000, -0.000000000000000000 ) ) ;
#40177=AXIS2_PLACEMENT_3D ( 'NONE', #28748, #42225, #7842 ) ;
#40201=EDGE_CURVE ( 'NONE', #20548, #41700, #22473, .T. ) ;
#40212=AXIS2_PLACEMENT_3D ( 'NONE', #25177, #34740, #15553 ) ;
#40215=CARTESIAN_POINT ( 'NONE',  ( 130.0000000000000284, 1.638195277402996435E-14, -20.00000000000000000 ) ) ;
#40253=ADVANCED_FACE ( 'NONE', ( #10496 ), #26655, .T. ) ;
#40275=AXIS2_PLACEMENT_3D ( 'NONE', #27582, #27813, #41065 ) ;
#40284=CARTESIAN_POINT ( 'NONE',  ( 0.000000000000000000, 0.000000000000000000, -25.00000000000000000 ) ) ;
#40327=AXIS2_PLACEMENT_3D ( 'NONE', #13889, #299, #36534 ) ;
#40350=ADVANCED_FACE ( 'NONE', ( #41673, #14660 ), #8081, .T. ) ;
#40366=DIRECTION ( 'NONE',  ( 0.000000000000000000, 0.000000000000000000, 1.000000000000000000 ) ) ;
#40371=EDGE_LOOP ( 'NONE', ( #13612, #42602 ) ) ;
#40408=EDGE_LOOP ( 'NONE', ( #20172, #6679, #11893, #30177 ) ) ;
#40459=ORIENTED_EDGE ( 'NONE', *, *, #36695, .F. ) ;
#40484=AXIS2_PLACEMENT_3D ( 'NONE', #34211, #37905, #34421 ) ;
#40540=EDGE_CURVE ( 'NONE', #11261, #21531, #1475, .T. ) ;
#40550=EDGE_CURVE ( 'NONE', #20273, #27122, #41879, .T. ) ;
#40559=ORIENTED_EDGE ( 'NONE', *, *, #21357, .T. ) ;
#40561=VERTEX_POINT ( 'NONE', #32496 ) ;
#40567=CARTESIAN_POINT ( 'NONE',  ( 5.657435538624008755E-15, 4.615443851143735910E-16, 0.000000000000000000 ) ) ;
#40574=EDGE_CURVE ( 'NONE', #40561, #2965, #25204, .T. ) ;
#40577=DIRECTION ( 'NONE',  ( -0.000000000000000000, -0.000000000000000000, 1.000000000000000000 ) ) ;
#40595=DIRECTION ( 'NONE',  ( 1.000000000000000000, 0.000000000000000000, 0.000000000000000000 ) ) ;
#40618=FACE_BOUND ( 'NONE', #23672, .T. ) ;
#40627=PLANE ( 'NONE',  #11740 ) ;
#40649=ORIENTED_EDGE ( 'NONE', *, *, #6217, .F. ) ;
#40657=EDGE_LOOP ( 'NONE', ( #2173, #16566 ) ) ;
#40689=ORIENTED_EDGE ( 'NONE', *, *, #40201, .T. ) ;
#40701=AXIS2_PLACEMENT_3D ( 'NONE', #14601, #37042, #23988 ) ;
#40757=DIRECTION ( 'NONE',  ( -0.000000000000000000, -0.000000000000000000, -1.000000000000000000 ) ) ;
#40869=LINE ( 'NONE', #37605, #36687 ) ;
#40870=CYLINDRICAL_SURFACE ( 'NONE', #35921, 2.649999999999999467 ) ;
#40914=EDGE_CURVE ( 'NONE', #22117, #28016, #25900, .T. ) ;
#40936=EDGE_CURVE ( 'NONE', #36435, #38324, #18979, .T. ) ;
#40964=ORIENTED_EDGE ( 'NONE', *, *, #23420, .T. ) ;
#40990=CARTESIAN_POINT ( 'NONE',  ( -103.7695705685748635, -106.4195705685759776, 9.999999999999998224 ) ) ;
#40999=DIRECTION ( 'NONE',  ( 1.000000000000000000, 0.000000000000000000, 0.000000000000000000 ) ) ;
#41065=DIRECTION ( 'NONE',  ( -1.000000000000000000, 0.000000000000000000, 0.000000000000000000 ) ) ;
#41138=EDGE_CURVE ( 'NONE', #14755, #7826, #41204, .T. ) ;
#41167=CIRCLE ( 'NONE', #36309, 126.0000000000000284 ) ;
#41204=CIRCLE ( 'NONE', #22456, 23.00000000000000000 ) ;
#41230=ADVANCED_FACE ( 'NONE', ( #36722 ), #14067, .F. ) ;
#41239=VERTEX_POINT ( 'NONE', #7051 ) ;
#41285=ORIENTED_EDGE ( 'NONE', *, *, #30147, .T. ) ;
#41293=VERTEX_POINT ( 'NONE', #41500 ) ;
#41302=DIRECTION ( 'NONE',  ( -0.000000000000000000, -0.000000000000000000, 1.000000000000000000 ) ) ;
#41396=CARTESIAN_POINT ( 'NONE',  ( 0.000000000000000000, 0.000000000000000000, -6.000000000000000000 ) ) ;
#41415=ORIENTED_EDGE ( 'NONE', *, *, #75, .F. ) ;
#41500=CARTESIAN_POINT ( 'NONE',  ( 158.5000000000000284, 0.000000000000000000, 6.999999999999998224 ) ) ;
#41533=CIRCLE ( 'NONE', #18585, 158.5000000000000284 ) ;
#41544=CYLINDRICAL_SURFACE ( 'NONE', #10979, 2.649999999999993694 ) ;
#41584=CARTESIAN_POINT ( 'NONE',  ( -23.00000000000000000, 0.000000000000000000, -6.000000000000000000 ) ) ;
#41617=CARTESIAN_POINT ( 'NONE',  ( 0.000000000000000000, 0.000000000000000000, -20.00000000000000000 ) ) ;
#41626=EDGE_LOOP ( 'NONE', ( #12329, #34364 ) ) ;
#41640=DIRECTION ( 'NONE',  ( -0.000000000000000000, -0.000000000000000000, 1.000000000000000000 ) ) ;
#41673=FACE_BOUND ( 'NONE', #34573, .T. ) ;
#41687=EDGE_CURVE ( 'NONE', #27790, #5016, #27346, .T. ) ;
#41700=VERTEX_POINT ( 'NONE', #36889 ) ;
#41759=EDGE_LOOP ( 'NONE', ( #22880, #19361, #15579, #37565 ) ) ;
#41765=CARTESIAN_POINT ( 'NONE',  ( 0.000000000000000000, 0.000000000000000000, 9.999999999999998224 ) ) ;
#41786=EDGE_CURVE ( 'NONE', #30139, #23467, #1567, .T. ) ;
#41797=CARTESIAN_POINT ( 'NONE',  ( -153.1500000000000057, -5.251434100941175950E-13, 6.999999999999998224 ) ) ;
#41811=DIRECTION ( 'NONE',  ( 0.000000000000000000, 0.000000000000000000, 1.000000000000000000 ) ) ;
#41879=LINE ( 'NONE', #42302, #10551 ) ;
#41902=CYLINDRICAL_SURFACE ( 'NONE', #23986, 2.649999999999985700 ) ;
#41920=ORIENTED_EDGE ( 'NONE', *, *, #7382, .F. ) ;
#41961=FACE_OUTER_BOUND ( 'NONE', #35214, .T. ) ;
#41980=CARTESIAN_POINT ( 'NONE',  ( 0.000000000000000000, 0.000000000000000000, 6.999999999999998224 ) ) ;
#41995=ADVANCED_FACE ( 'NONE', ( #35746 ), #35549, .F. ) ;
#42050=CYLINDRICAL_SURFACE ( 'NONE', #6004, 2.649999999999985700 ) ;
#42053=AXIS2_PLACEMENT_3D ( 'NONE', #8090, #18830, #1748 ) ;
#42061=DIRECTION ( 'NONE',  ( 1.000000000000000000, 0.000000000000000000, 0.000000000000000000 ) ) ;
#42115=ORIENTED_EDGE ( 'NONE', *, *, #24368, .F. ) ;
#42140=ORIENTED_EDGE ( 'NONE', *, *, #9490, .T. ) ;
#42178=CIRCLE ( 'NONE', #38018, 126.0000000000000284 ) ;
#42188=DIRECTION ( 'NONE',  ( 1.000000000000000000, 0.000000000000000000, 0.000000000000000000 ) ) ;
#42197=VECTOR ( 'NONE', #17572, 1000.000000000000000 ) ;
#42214=AXIS2_PLACEMENT_3D ( 'NONE', #40567, #11362, #10938 ) ;
#42225=DIRECTION ( 'NONE',  ( 0.000000000000000000, 0.000000000000000000, 1.000000000000000000 ) ) ;
#42261=ADVANCED_FACE ( 'NONE', ( #38141 ), #8264, .T. ) ;
#42285=CARTESIAN_POINT ( 'NONE',  ( -106.4195705685756081, 106.4195705685752529, 9.999999999999998224 ) ) ;
#42295=DIRECTION ( 'NONE',  ( 1.000000000000000000, 0.000000000000000000, 0.000000000000000000 ) ) ;
#42302=CARTESIAN_POINT ( 'NONE',  ( -12.50000000000000000, 1.530808498934191521E-15, -25.00000000000000000 ) ) ;
#42367=EDGE_LOOP ( 'NONE', ( #10917, #19231, #3546, #25876 ) ) ;
#42451=CIRCLE ( 'NONE', #15933, 130.0000000000000000 ) ;
#42513=DIRECTION ( 'NONE',  ( 0.000000000000000000, 0.000000000000000000, 1.000000000000000000 ) ) ;
#42602=ORIENTED_EDGE ( 'NONE', *, *, #30147, .F. ) ;
#42624=AXIS2_PLACEMENT_3D ( 'NONE', #17333, #675, #40595 ) ;
#42722=DIRECTION ( 'NONE',  ( 0.000000000000000000, 0.000000000000000000, 1.000000000000000000 ) ) ;
#42755=ORIENTED_EDGE ( 'NONE', *, *, #31626, .T. ) ;
#42866=FACE_BOUND ( 'NONE', #14101, .T. ) ;
#42896=VECTOR ( 'NONE', #41302, 1000.000000000000000 ) ;
#42908=DIRECTION ( 'NONE',  ( -0.000000000000000000, -0.000000000000000000, 1.000000000000000000 ) ) ;
#42940=DIRECTION ( 'NONE',  ( 0.000000000000000000, 0.000000000000000000, 1.000000000000000000 ) ) ;
#42959=VECTOR ( 'NONE', #35446, 1000.000000000000000 ) ;
#42992=EDGE_CURVE ( 'NONE', #15086, #32065, #6207, .T. ) ;
#42996=FACE_OUTER_BOUND ( 'NONE', #9823, .T. ) ;
#43017=DIRECTION ( 'NONE',  ( -0.000000000000000000, -0.000000000000000000, -1.000000000000000000 ) ) ;
#43123=DIRECTION ( 'NONE',  ( 1.000000000000000000, 0.000000000000000000, 0.000000000000000000 ) ) ;
#43131=CARTESIAN_POINT ( 'NONE',  ( -23.00000000000000000, 0.000000000000000000, -6.000000000000000000 ) ) ;
#43154=DIRECTION ( 'NONE',  ( 1.000000000000000000, 0.000000000000000000, 0.000000000000000000 ) ) ;
ENDSEC;
END-ISO-10303-21;
